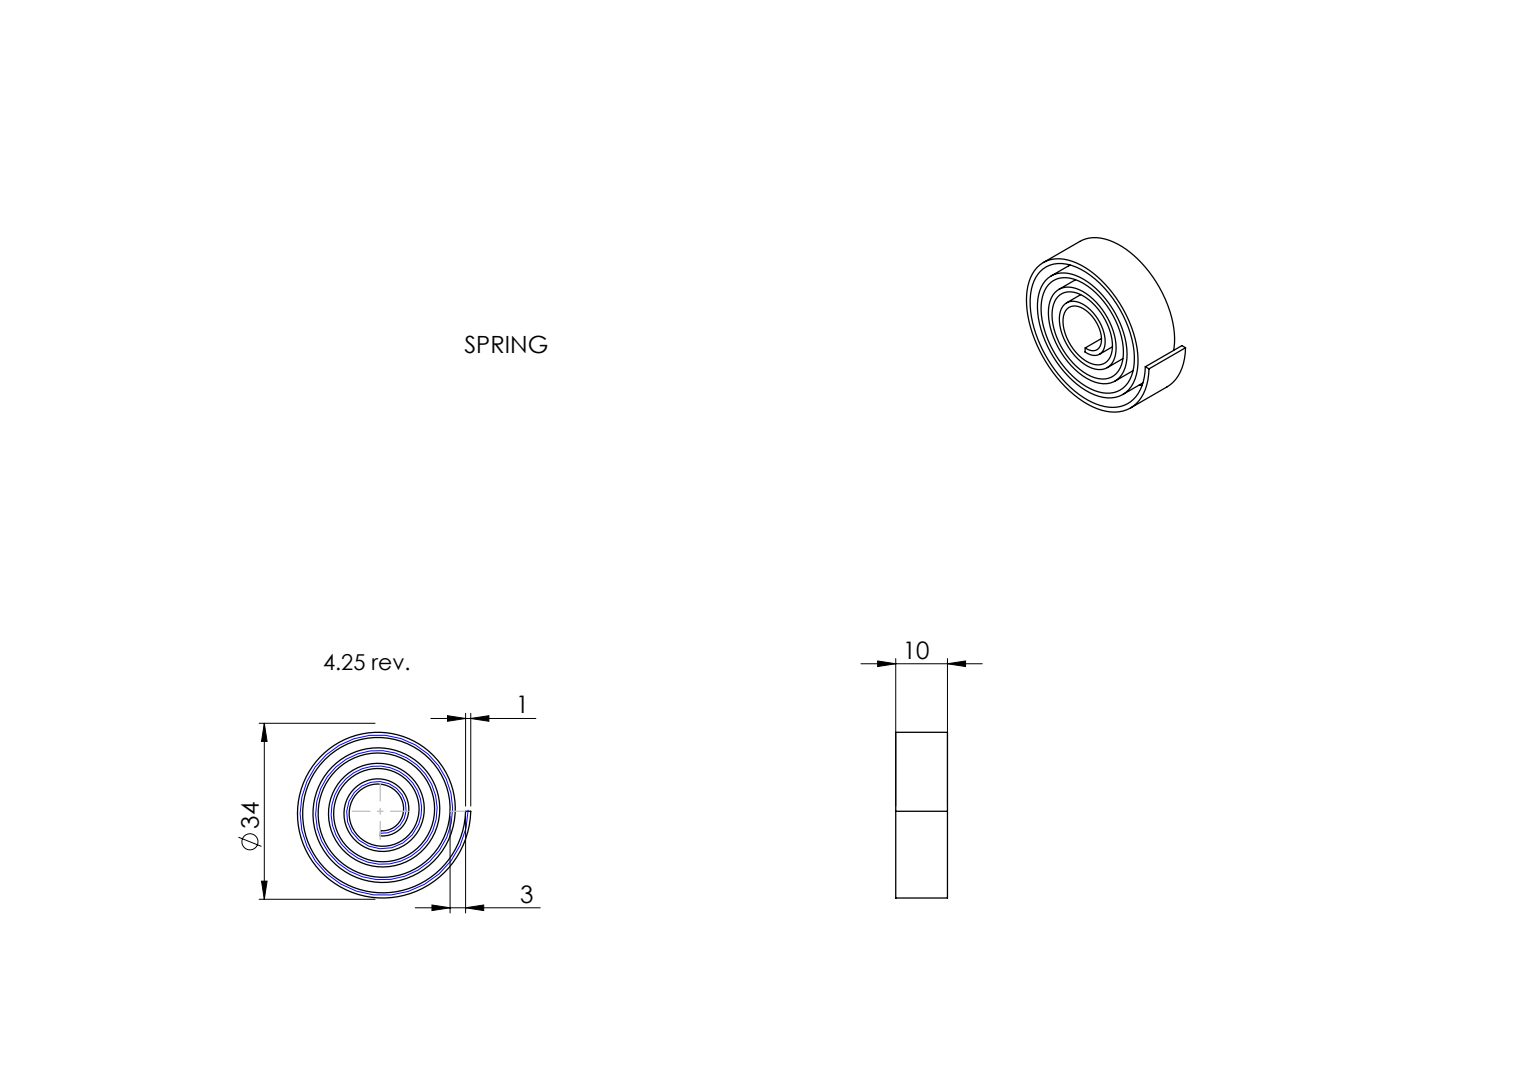
ISO-10303-21;
HEADER;
FILE_DESCRIPTION (('STEP AP214'),
    '1' );
FILE_NAME ('spring.step',
    '2026-10-08T12:30:53',
    ( '' ),
    ( '' ),
    'SwSTEP 2.0',
    'SolidWorks 2026',
    '' );
FILE_SCHEMA (( 'AUTOMOTIVE_DESIGN' ));
ENDSEC;

DATA;
#5=CARTESIAN_POINT ( 'NONE',  ( 13.54728169684850414, 0.8932250400876640128, 10.00000000000000000 ) ) ;
#11=CARTESIAN_POINT ( 'NONE',  ( -13.43906451854578954, -9.301052350413227643, 10.00000000000000000 ) ) ;
#12=CARTESIAN_POINT ( 'NONE',  ( 8.539395351299290837, 0.2748098766782898217, 6.857782953271941950E-17 ) ) ;
#18=PRODUCT ( 'spring', 'spring', '', ( #10456 ) ) ;
#19=EDGE_LOOP ( 'NONE', ( #9760, #9661, #8021, #4048 ) ) ;
#26=CARTESIAN_POINT ( 'NONE',  ( 10.50580257846854337, 1.391709641844861123, 10.00000000000000000 ) ) ;
#31=CARTESIAN_POINT ( 'NONE',  ( 8.800885721068835821, 6.316044917328127895, 3.747395293195558847E-16 ) ) ;
#46=CARTESIAN_POINT ( 'NONE',  ( -11.99326810842395474, 8.590522060507202795, 3.747395293195558847E-16 ) ) ;
#63=CARTESIAN_POINT ( 'NONE',  ( -6.211147023100844322, 2.816369743025010308, 10.00000000000000000 ) ) ;
#73=CARTESIAN_POINT ( 'NONE',  ( 12.88139461472802516, -9.891864711285373701, 10.00000000000000000 ) ) ;
#78=CARTESIAN_POINT ( 'NONE',  ( -3.251399079312189855, 15.05603916236422890, 10.00000000000000000 ) ) ;
#79=CARTESIAN_POINT ( 'NONE',  ( 5.267519402444978738, 2.381954139586884622, 6.857782953271941950E-17 ) ) ;
#88=CARTESIAN_POINT ( 'NONE',  ( -8.694522232909452697, -2.966707450564700643, 10.00000000000000000 ) ) ;
#91=CARTESIAN_POINT ( 'NONE',  ( 9.962304844536467030, 3.945508033568876360, 3.747395293195558847E-16 ) ) ;
#105=CARTESIAN_POINT ( 'NONE',  ( 1.050035089571674352, -12.78847817906846096, 3.747395293195558847E-16 ) ) ;
#109=ORIENTED_EDGE ( 'NONE', *, *, #7807, .F. ) ;
#111=CARTESIAN_POINT ( 'NONE',  ( -10.11701526667144257, 11.92482893257633947, 10.00000000000000000 ) ) ;
#120=CARTESIAN_POINT ( 'NONE',  ( -12.27443204883033623, 3.949650873796764827, 6.857782953271941950E-17 ) ) ;
#127=CARTESIAN_POINT ( 'NONE',  ( -3.043536693350107569, 14.07442491708026111, 10.00000000000000000 ) ) ;
#131=CARTESIAN_POINT ( 'NONE',  ( 10.35108484788239203, -9.702746953904565430, 10.00000000000000000 ) ) ;
#142=CARTESIAN_POINT ( 'NONE',  ( -8.962830026514758686, 0.7152994853347287574, 10.00000000000000000 ) ) ;
#146=CARTESIAN_POINT ( 'NONE',  ( -0.1586286459269546645, 8.284426055182338544, 3.747395293195558847E-16 ) ) ;
#147=CARTESIAN_POINT ( 'NONE',  ( -14.12277927129995803, -8.146689865454474599, 6.857782953271941950E-17 ) ) ;
#160=CARTESIAN_POINT ( 'NONE',  ( 4.123629756449401107, -15.38522696314584515, 3.747395293195558847E-16 ) ) ;
#161=B_SPLINE_CURVE_WITH_KNOTS ( 'NONE', 3,
 ( #5386, #11258, #9477, #10271, #12042, #10215, #12099, #7452, #5566, #5686, #3851, #160, #7515, #4646, #6654, #11313, #9416, #9236, #7383, #10392, #2746, #1763, #2872, #3726, #5623, #6594, #5504, #8321, #3906, #856, #2009, #46, #11199, #4589, #1040, #5753, #1094, #913, #4825, #7630, #10329, #8563, #2815, #11374, #6539, #2994, #9353, #6716, #3663, #11126, #7571, #6477, #4770, #1830, #9296, #3796, #1889, #970, #8381, #4710, #8449, #1947, #8509, #2933, #105, #5808, #11490, #10452, #2070, #5004, #9535, #1151, #7935, #4206, #2189, #4887, #8625, #2303, #3969, #3113, #8687, #225, #10574, #5125, #8800, #6946, #5984, #7698, #11433, #6039, #1391, #1325, #4087, #10690, #4024, #9597, #3053, #3228, #6772, #10509, #9711, #1215, #9768, #2124, #5062, #8863, #11664, #408, #7880, #5865, #4951, #3282, #6828, #5928, #468, #286, #7753, #9657, #1271, #4153, #8742, #2249, #11611, #345, #7815, #11553, #3175, #6894, #10638, #8975, #3350, #11847, #7002, #11906, #8058, #9153, #10749, #585, #7066, #6106, #3533, #7247, #11790, #770, #2367, #4324, #10820, #9840, #11001, #2551, #1450, #528, #2615, #7987, #11723, #8178, #11967, #4444, #2429, #3420, #4261, #4507, #5185, #6350, #5309, #7127, #8920, #10933, #10073, #1692, #6167, #5425, #8243, #4388, #10877, #9895, #7186, #1508, #5243, #2488, #6225, #9952, #1569, #9100, #9042, #6290, #655, #8121, #3476, #10010, #1636, #5374, #710, #8306, #12028, #6526, #1933, #2735, #5669, #3652, #6463, #3595, #7435, #11056, #2671, #7560, #3838, #4633 ),
 .UNSPECIFIED., .F., .F.,
 ( 4, 2, 2, 2, 2, 2, 2, 2, 2, 2, 2, 2, 2, 2, 2, 2, 2, 2, 2, 2, 2, 2, 2, 2, 2, 2, 2, 2, 2, 2, 2, 2, 2, 2, 2, 2, 2, 2, 2, 2, 2, 2, 2, 2, 2, 2, 2, 2, 2, 2, 2, 2, 2, 2, 2, 2, 2, 2, 2, 2, 2, 2, 2, 2, 2, 2, 2, 2, 2, 2, 2, 2, 2, 2, 2, 2, 2, 2, 2, 2, 2, 2, 2, 2, 2, 2, 2, 2, 2, 2, 2, 2, 2, 2, 2, 2, 2, 2, 2, 2, 2, 2, 2, 4 ),
 ( 0.000000000000000000, 0.007812500000000000000, 0.01562500000000000000, 0.02343750000000000000, 0.03125000000000000000, 0.03906250000000000000, 0.04687500000000000000, 0.05468750000000000000, 0.06250000000000000000, 0.07031250000000000000, 0.07812500000000000000, 0.08593750000000000000, 0.09375000000000000000, 0.1015624999999999861, 0.1093750000000000000, 0.1171875000000000000, 0.1250000000000000000, 0.1328125000000000000, 0.1406250000000000000, 0.1484375000000000000, 0.1562500000000000000, 0.1640624999999999722, 0.1718750000000000000, 0.1796875000000000000, 0.1875000000000000000, 0.1953125000000000000, 0.2031249999999999722, 0.2109375000000000000, 0.2187500000000000000, 0.2265625000000000000, 0.2343750000000000000, 0.2421875000000000000, 0.2500000000000000000, 0.2578125000000000000, 0.2656250000000000000, 0.2734375000000000000, 0.2812500000000000000, 0.2890625000000000000, 0.2968750000000000000, 0.3046875000000000000, 0.3125000000000000000, 0.3203125000000000000, 0.3281249999999999445, 0.3359375000000000000, 0.3437500000000000000, 0.3515625000000000000, 0.3593750000000000000, 0.3671874999999999445, 0.3750000000000000000, 0.3828125000000000000, 0.3906250000000000000, 0.3984375000000000000, 0.4062499999999999445, 0.4140625000000000000, 0.4218750000000000000, 0.4296875000000000000, 0.4375000000000000000, 0.4453125000000000000, 0.4531250000000000000, 0.4609375000000000000, 0.4687500000000000000, 0.4765625000000000000, 0.4843750000000000000, 0.4921875000000000000, 0.5000000000000000000, 0.5078125000000000000, 0.5156250000000000000, 0.5234375000000000000, 0.5312500000000000000, 0.5390625000000000000, 0.5468750000000000000, 0.5546875000000000000, 0.5625000000000000000, 0.5703125000000000000, 0.5781250000000000000, 0.5859375000000000000, 0.5937500000000000000, 0.6015625000000000000, 0.6093750000000000000, 0.6171874999999998890, 0.6250000000000000000, 0.6328125000000000000, 0.6406250000000000000, 0.6484375000000000000, 0.6562499999999998890, 0.6640625000000000000, 0.6718750000000000000, 0.6796875000000000000, 0.6875000000000000000, 0.6953124999999998890, 0.7031250000000000000, 0.7109375000000000000, 0.7187500000000000000, 0.7265625000000000000, 0.7343749999999998890, 0.7421875000000000000, 0.7500000000000000000, 0.7656250000000000000, 0.7812500000000000000, 0.7968750000000000000, 0.8124999999999998890, 0.8281250000000000000, 0.8437500000000000000, 0.8499999999999999778 ),
 .UNSPECIFIED. ) ;
#167=CARTESIAN_POINT ( 'NONE',  ( -12.80690425020244128, 9.177692349400032867, 10.00000000000000000 ) ) ;
#177=CARTESIAN_POINT ( 'NONE',  ( -10.84705874452746066, 6.751620637727320684, 6.857782953271941950E-17 ) ) ;
#185=CARTESIAN_POINT ( 'NONE',  ( -15.00596061316374197, -1.728743269517114767, 10.00000000000000000 ) ) ;
#191=CARTESIAN_POINT ( 'NONE',  ( 14.53830338343600559, -0.2437330612273629071, 10.00000000000000000 ) ) ;
#202=CARTESIAN_POINT ( 'NONE',  ( 2.581500635392915299, -6.456130005640037695, 10.00000000000000000 ) ) ;
#206=CARTESIAN_POINT ( 'NONE',  ( 7.605204090344414247, 4.385345779697003010, 10.00000000000000000 ) ) ;
#208=CARTESIAN_POINT ( 'NONE',  ( -12.06849956494802889, -5.462025159506374017, 6.857782953271941950E-17 ) ) ;
#213=EDGE_CURVE ( 'NONE', #1474, #6584, #2468, .T. ) ;
#225=CARTESIAN_POINT ( 'NONE',  ( -10.51222845931327576, 5.388985543800765221, 3.747395293195558847E-16 ) ) ;
#233=CARTESIAN_POINT ( 'NONE',  ( 4.382127860174852785, -16.35473703246191235, 10.00000000000000000 ) ) ;
#244=CARTESIAN_POINT ( 'NONE',  ( 5.334478431285537781, 14.15651896542076749, 6.857782953271941950E-17 ) ) ;
#252=CARTESIAN_POINT ( 'NONE',  ( -4.793139000956300855, -14.90149022103883247, 10.00000000000000000 ) ) ;
#259=CARTESIAN_POINT ( 'NONE',  ( 7.737545192982512532, 9.111483571581279861, 10.00000000000000000 ) ) ;
#262=CARTESIAN_POINT ( 'NONE',  ( -6.423942855642367000, 13.01866063961475461, 3.747395293195558847E-16 ) ) ;
#270=CARTESIAN_POINT ( 'NONE',  ( 1.482756436301465808, -6.713508106970953015, 10.00000000000000000 ) ) ;
#272=CARTESIAN_POINT ( 'NONE',  ( 11.51680056346192593, -0.3781118375584788249, 10.00000000000000000 ) ) ;
#273=CARTESIAN_POINT ( 'NONE',  ( 1.748316258820581170, 15.14524454193558611, 6.857782953271941950E-17 ) ) ;
#281=CARTESIAN_POINT ( 'NONE',  ( 3.017784444055084503, -16.62017357425735753, 6.857782953271941950E-17 ) ) ;
#286=CARTESIAN_POINT ( 'NONE',  ( 0.6578947103914138950, -9.792230064638470566, 3.747395293195558847E-16 ) ) ;
#293=CARTESIAN_POINT ( 'NONE',  ( -15.56595607421884075, -4.438723023272252988, 10.00000000000000000 ) ) ;
#305=CARTESIAN_POINT ( 'NONE',  ( -3.251399079312188078, 15.05603916236422180, 6.857782953271941950E-17 ) ) ;
#312=CARTESIAN_POINT ( 'NONE',  ( 4.071483724746832067, 10.33449570568845211, 10.00000000000000000 ) ) ;
#314=( NAMED_UNIT ( * ) PLANE_ANGLE_UNIT ( ) SI_UNIT ( $, .RADIAN. ) );
#317=CARTESIAN_POINT ( 'NONE',  ( 12.58137556868281237, 7.823023050435613968, 10.00000000000000000 ) ) ;
#329=CARTESIAN_POINT ( 'NONE',  ( -0.7379871813790722657, -6.677365878963855472, 10.00000000000000000 ) ) ;
#333=CARTESIAN_POINT ( 'NONE',  ( -8.201440678128605555, 5.289679325232168772, 10.00000000000000000 ) ) ;
#334=CARTESIAN_POINT ( 'NONE',  ( -15.59049818040117152, 3.373450308083002724, 6.857782953271941950E-17 ) ) ;
#342=CARTESIAN_POINT ( 'NONE',  ( 7.795318149608632119, -14.02504990430958998, 10.00000000000000000 ) ) ;
#345=CARTESIAN_POINT ( 'NONE',  ( -7.402161455537873636, -5.702533393948970186, 3.747395293195558847E-16 ) ) ;
#349=CARTESIAN_POINT ( 'NONE',  ( 17.46093749967478814, -1.431715403549062904, 10.00000000000000000 ) ) ;
#352=VECTOR ( 'NONE', #8492, 1000.000000000000000 ) ;
#359=CARTESIAN_POINT ( 'NONE',  ( -2.240087900411201982, -13.53314956822677928, 6.857782953271941950E-17 ) ) ;
#369=CARTESIAN_POINT ( 'NONE',  ( -4.046710180314750716, 10.72208681399755648, 10.00000000000000000 ) ) ;
#377=CARTESIAN_POINT ( 'NONE',  ( 2.259453438922059298, -13.68937604509904737, 10.00000000000000000 ) ) ;
#379=CARTESIAN_POINT ( 'NONE',  ( -11.21689850597007343, 9.520844388990626683, 3.747395293195558847E-16 ) ) ;
#391=CARTESIAN_POINT ( 'NONE',  ( -6.589974825828277538, 7.038139701356666222, 10.00000000000000000 ) ) ;
#393=CARTESIAN_POINT ( 'NONE',  ( -12.72059027619867244, -3.407653011835690471, 6.857782953271941950E-17 ) ) ;
#408=CARTESIAN_POINT ( 'NONE',  ( 8.913847851857145344, -5.129921849437907078, 3.747395293195558847E-16 ) ) ;
#413=CARTESIAN_POINT ( 'NONE',  ( -8.799721882313775723, 9.100398320382247164, 10.00000000000000000 ) ) ;
#424=CARTESIAN_POINT ( 'NONE',  ( -9.352287007201468327, 3.176141031410556703, 6.857782953271941950E-17 ) ) ;
#430=CARTESIAN_POINT ( 'NONE',  ( -8.984113827416489784, -1.502549133976348816, 10.00000000000000000 ) ) ;
#439=CARTESIAN_POINT ( 'NONE',  ( 3.343943643650761022, -10.41127694127790271, 10.00000000000000000 ) ) ;
#454=CARTESIAN_POINT ( 'NONE',  ( 5.893263639827395650, 6.717612500730409941, 10.00000000000000000 ) ) ;
#456=CARTESIAN_POINT ( 'NONE',  ( 5.343773788080180331, 10.82393792025543711, 6.857782953271941950E-17 ) ) ;
#468=CARTESIAN_POINT ( 'NONE',  ( 2.257301671556970479, -9.631158585656898197, 3.747395293195558847E-16 ) ) ;
#473=CARTESIAN_POINT ( 'NONE',  ( 14.27634331491212549, 3.322769473269123974, 10.00000000000000000 ) ) ;
#485=CARTESIAN_POINT ( 'NONE',  ( -8.201440678127905670, 5.289679325232165219, 6.857782953271941950E-17 ) ) ;
#491=CARTESIAN_POINT ( 'NONE',  ( -10.00031051369627200, 6.213292778947749007, 10.00000000000000000 ) ) ;
#498=CARTESIAN_POINT ( 'NONE',  ( -4.368568794346924022, -9.638580752213403713, 10.00000000000000000 ) ) ;
#500=CARTESIAN_POINT ( 'NONE',  ( -11.74902089294173457, -3.156991809147609906, 3.747395293195558847E-16 ) ) ;
#513=CARTESIAN_POINT ( 'NONE',  ( 2.919619825260427071, -7.400844473264730716, 10.00000000000000000 ) ) ;
#514=CARTESIAN_POINT ( 'NONE',  ( -3.909826107002860596, 8.641065831729461522, 6.857782953271941950E-17 ) ) ;
#522=CARTESIAN_POINT ( 'NONE',  ( -15.00596061316374197, -1.728743269517114767, 10.00000000000000000 ) ) ;
#528=CARTESIAN_POINT ( 'NONE',  ( 7.195390336726608105, 2.736402267197653337, 3.747395293195558847E-16 ) ) ;
#533=CARTESIAN_POINT ( 'NONE',  ( -11.61414229320030778, -6.453515506896109422, 10.00000000000000000 ) ) ;
#543=CARTESIAN_POINT ( 'NONE',  ( -3.909826107002860596, 8.641065831729461522, 6.857782953271941950E-17 ) ) ;
#550=CARTESIAN_POINT ( 'NONE',  ( 8.800885721068839374, 6.316044917328129671, 10.00000000000000000 ) ) ;
#558=CARTESIAN_POINT ( 'NONE',  ( 0.7062845326068618590, -10.79445016380499212, 10.00000000000000000 ) ) ;
#560=CARTESIAN_POINT ( 'NONE',  ( 7.972781652389871354, 11.51689705412852405, 3.747395293195558847E-16 ) ) ;
#575=CARTESIAN_POINT ( 'NONE',  ( 2.798030692818294085, 8.692477993603722197, 6.857782953271941950E-17 ) ) ;
#582=CARTESIAN_POINT ( 'NONE',  ( -14.24631147015002242, -5.364320868108786833, 10.00000000000000000 ) ) ;
#585=CARTESIAN_POINT ( 'NONE',  ( -4.158289900079266133, 7.437556212723415605, 3.747395293195558847E-16 ) ) ;
#595=CARTESIAN_POINT ( 'NONE',  ( -5.414455899168761022, -12.47541146649038879, 10.00000000000000000 ) ) ;
#608=CARTESIAN_POINT ( 'NONE',  ( -7.708066421255707290, 5.920849505456867945, 6.857782953271941950E-17 ) ) ;
#617=CARTESIAN_POINT ( 'NONE',  ( 5.657123057053187409, 5.504982807385219168, 10.00000000000000000 ) ) ;
#625=CARTESIAN_POINT ( 'NONE',  ( 7.252227276002106038, 5.017415995114419047, 10.00000000000000000 ) ) ;
#628=CARTESIAN_POINT ( 'NONE',  ( -1.035167565893234443, -12.71157708251009133, 3.747395293195558847E-16 ) ) ;
#640=CARTESIAN_POINT ( 'NONE',  ( 1.661435237661583297, -7.700870200009183542, 10.00000000000000000 ) ) ;
#641=CARTESIAN_POINT ( 'NONE',  ( -4.625218816436122538, 8.325684435358754243, 6.857782953271941950E-17 ) ) ;
#650=CARTESIAN_POINT ( 'NONE',  ( -2.069312577552833154, -12.54440658741724235, 10.00000000000000000 ) ) ;
#654=CARTESIAN_POINT ( 'NONE',  ( 0.03696586647634111239, -4.250492970015663730, 10.00000000000000000 ) ) ;
#655=CARTESIAN_POINT ( 'NONE',  ( -4.158472309566738190, 3.840014155104740201, 3.747395293195558847E-16 ) ) ;
#663=CARTESIAN_POINT ( 'NONE',  ( -1.784247137544766604, 5.123456263349899231, 10.00000000000000000 ) ) ;
#671=CARTESIAN_POINT ( 'NONE',  ( 10.96671743108978525, -3.132869264233209439, 6.857782953271941950E-17 ) ) ;
#677=CARTESIAN_POINT ( 'NONE',  ( 7.536008357046525497, 0.2705779428718255719, 10.00000000000000000 ) ) ;
#685=CARTESIAN_POINT ( 'NONE',  ( -0.2556890074706391625, -7.756263830888999067, 10.00000000000000000 ) ) ;
#692=CARTESIAN_POINT ( 'NONE',  ( 6.411932913580776550, 4.469049885107575726, 3.747395293195558847E-16 ) ) ;
#698=CARTESIAN_POINT ( 'NONE',  ( -6.211147023100844322, 2.816369743025010308, 10.00000000000000000 ) ) ;
#699=CARTESIAN_POINT ( 'NONE',  ( -8.665663522307772482, -5.581295667939712324, 6.857782953271941950E-17 ) ) ;
#706=CARTESIAN_POINT ( 'NONE',  ( -5.318373871714366707, 13.46535835423756566, 10.00000000000000000 ) ) ;
#710=CARTESIAN_POINT ( 'NONE',  ( -0.4771094043438768861, 5.286185534804329400, 3.747395293195558847E-16 ) ) ;
#724=CARTESIAN_POINT ( 'NONE',  ( 7.763517025772753044, -3.069710483245351451, 6.857782953271941950E-17 ) ) ;
#731=CARTESIAN_POINT ( 'NONE',  ( 6.723006375386864519, 3.907299473125435796, 10.00000000000000000 ) ) ;
#739=CARTESIAN_POINT ( 'NONE',  ( 17.46093749967478104, -1.431715403549062460, 6.857782953271941950E-17 ) ) ;
#746=ADVANCED_FACE ( 'NONE', ( #3811 ), #3925, .T. ) ;
#749=CARTESIAN_POINT ( 'NONE',  ( 0.8073695008816142993, 5.181225205791315958, 3.747395293195558847E-16 ) ) ;
#750=AXIS2_PLACEMENT_3D ( 'NONE', #910, #10269, #9233 ) ;
#756=CARTESIAN_POINT ( 'NONE',  ( 2.529667540517110513, -4.392173529266737653, 10.00000000000000000 ) ) ;
#757=CARTESIAN_POINT ( 'NONE',  ( 4.138106518798946531, 8.052838533163340529, 6.857782953271941950E-17 ) ) ;
#763=CARTESIAN_POINT ( 'NONE',  ( -8.499083411061075566, 11.86528080735166490, 10.00000000000000000 ) ) ;
#770=CARTESIAN_POINT ( 'NONE',  ( 1.831757423467612389, 7.960349185506225389, 3.747395293195558847E-16 ) ) ;
#794=CARTESIAN_POINT ( 'NONE',  ( 7.195390336726611658, 2.736402267197346028, 10.00000000000000000 ) ) ;
#803=CARTESIAN_POINT ( 'NONE',  ( 3.017784444055084503, -16.62017357425735753, 6.857782953271941950E-17 ) ) ;
#809=ORIENTED_EDGE ( 'NONE', *, *, #6284, .T. ) ;
#813=CARTESIAN_POINT ( 'NONE',  ( 7.527773320476327079, 0.8933511214758176333, 3.747395293195558847E-16 ) ) ;
#822=CARTESIAN_POINT ( 'NONE',  ( 2.529667540516381319, -4.392173529266732324, 6.857782953271941950E-17 ) ) ;
#832=CARTESIAN_POINT ( 'NONE',  ( -10.00031051369627200, 6.213292778947749007, 10.00000000000000000 ) ) ;
#838=CARTESIAN_POINT ( 'NONE',  ( -3.937910939466568117, -8.732312745279397603, 3.747395293195558847E-16 ) ) ;
#852=UNCERTAINTY_MEASURE_WITH_UNIT (LENGTH_MEASURE( 1.000000000000000082E-05 ), #3873, 'distance_accuracy_value', 'NONE');
#856=CARTESIAN_POINT ( 'NONE',  ( -13.83044629298881034, 5.462350471645222250, 3.747395293195558847E-16 ) ) ;
#857=CARTESIAN_POINT ( 'NONE',  ( 8.393308867179008814, -1.106660293010312213, 6.857782953271941950E-17 ) ) ;
#865=CARTESIAN_POINT ( 'NONE',  ( -3.432991321284830200, 4.402131891631372973, 10.00000000000000000 ) ) ;
#872=CARTESIAN_POINT ( 'NONE',  ( -5.542557460684662374, -4.854674288180239827, 10.00000000000000000 ) ) ;
#880=CARTESIAN_POINT ( 'NONE',  ( -0.7379871813790714885, -6.677365878963852808, 3.747395293195558847E-16 ) ) ;
#885=CARTESIAN_POINT ( 'NONE',  ( 4.382127860174852785, -16.35473703246191235, 10.00000000000000000 ) ) ;
#886=CARTESIAN_POINT ( 'NONE',  ( 0.3111040546027372677, -4.780743156735971944, 6.857782953271941950E-17 ) ) ;
#892=CARTESIAN_POINT ( 'NONE',  ( 4.071483724746832067, 10.33449570568845211, 10.00000000000000000 ) ) ;
#897=CARTESIAN_POINT ( 'NONE',  ( 10.00611923916670953, -2.842981073525689517, 3.747395293195558847E-16 ) ) ;
#910=CARTESIAN_POINT ( 'NONE',  ( 17.49999999999999645, 0.000000000000000000, 6.857782953271941950E-17 ) ) ;
#913=CARTESIAN_POINT ( 'NONE',  ( -3.043536693350106681, 14.07442491708025756, 3.747395293195558847E-16 ) ) ;
#914=CARTESIAN_POINT ( 'NONE',  ( -6.191802569540376666, -3.848120238389427072, 6.857782953271941950E-17 ) ) ;
#926=CARTESIAN_POINT ( 'NONE',  ( -4.263796145714478847, -6.152586724582791433, 10.00000000000000000 ) ) ;
#936=CARTESIAN_POINT ( 'NONE',  ( -4.158472309566738190, 3.840014155104740201, 3.747395293195558847E-16 ) ) ;
#942=CARTESIAN_POINT ( 'NONE',  ( 17.24531215409499296, -2.853661713830125013, 10.00000000000000000 ) ) ;
#943=CARTESIAN_POINT ( 'NONE',  ( 5.893263639826756162, 6.717612500731040548, 6.857782953271941950E-17 ) ) ;
#951=CARTESIAN_POINT ( 'NONE',  ( 10.39479819782869896, 2.258419626871297492, 10.00000000000000000 ) ) ;
#955=CARTESIAN_POINT ( 'NONE',  ( 1.454091968623351327, 11.13059540125182423, 3.747395293195558847E-16 ) ) ;
#970=CARTESIAN_POINT ( 'NONE',  ( 10.36190401370965475, -8.216093097539266310, 3.747395293195558847E-16 ) ) ;
#971=CARTESIAN_POINT ( 'NONE',  ( 1.022653496104248605, 6.171874473422422902, 6.857782953271941950E-17 ) ) ;
#989=CARTESIAN_POINT ( 'NONE',  ( 17.24531215409252383, -2.853661713830123237, 6.857782953271941950E-17 ) ) ;
#990=CARTESIAN_POINT ( 'NONE',  ( 0.0002901587068754535662, -4.749354241797641762, 5.000000000000000000 ) ) ;
#999=CARTESIAN_POINT ( 'NONE',  ( 4.163410377374356486, -12.26152398776834396, 10.00000000000000000 ) ) ;
#1008=CARTESIAN_POINT ( 'NONE',  ( -6.864300873105356082, 13.92024697337932082, 10.00000000000000000 ) ) ;
#1009=CARTESIAN_POINT ( 'NONE',  ( -6.211147023100837217, 2.816369743025007644, 6.857782953271941950E-17 ) ) ;
#1021=CARTESIAN_POINT ( 'NONE',  ( -10.51222845931418703, 5.388985543801221745, 10.00000000000000000 ) ) ;
#1024=CARTESIAN_POINT ( 'NONE',  ( -6.925491926711623059, 5.292860106065907289, 3.747395293195558847E-16 ) ) ;
#1040=CARTESIAN_POINT ( 'NONE',  ( -8.499083411061073789, 11.86528080735276269, 3.747395293195558847E-16 ) ) ;
#1045=CARTESIAN_POINT ( 'NONE',  ( -1.103316172498668202, -16.73802372459124754, 10.00000000000000000 ) ) ;
#1053=CARTESIAN_POINT ( 'NONE',  ( 4.479449988082533807, -13.21383449271837840, 6.857782953271941950E-17 ) ) ;
#1062=CARTESIAN_POINT ( 'NONE',  ( -6.423942855642368777, 13.01866063961585951, 10.00000000000000000 ) ) ;
#1069=CARTESIAN_POINT ( 'NONE',  ( -4.384918567263696332, -12.91535881965571342, 10.00000000000000000 ) ) ;
#1077=CARTESIAN_POINT ( 'NONE',  ( 10.41236255589547177, -1.188820951657899361, 10.00000000000000000 ) ) ;
#1079=CARTESIAN_POINT ( 'NONE',  ( -8.409270314015810044, 2.833341551407462244, 3.747395293195558847E-16 ) ) ;
#1080=CARTESIAN_POINT ( 'NONE',  ( -14.19814495527598730, 7.008511237308412412, 6.857782953271941950E-17 ) ) ;
#1094=CARTESIAN_POINT ( 'NONE',  ( -5.318373871714365819, 13.46535835423756389, 3.747395293195558847E-16 ) ) ;
#1107=CARTESIAN_POINT ( 'NONE',  ( -9.546882484473291797, 8.373557015400844961, 6.857782953271941950E-17 ) ) ;
#1114=CARTESIAN_POINT ( 'NONE',  ( 11.62709622633371076, -6.461356448465072511, 10.00000000000000000 ) ) ;
#1121=CARTESIAN_POINT ( 'NONE',  ( -6.266017822847497420, 10.86399168115691438, 10.00000000000000000 ) ) ;
#1123=CARTESIAN_POINT ( 'NONE',  ( -14.24631147015001886, -5.364320868109360596, 3.747395293195558847E-16 ) ) ;
#1133=CARTESIAN_POINT ( 'NONE',  ( 7.402789038520873000, -0.9464297003978345835, 10.00000000000000000 ) ) ;
#1135=CARTESIAN_POINT ( 'NONE',  ( -9.977213461302319786, -1.645879626164742593, 10.00000000000000000 ) ) ;
#1137=CARTESIAN_POINT ( 'NONE',  ( -4.384918567263694555, -12.91535881965570631, 6.857782953271941950E-17 ) ) ;
#1151=CARTESIAN_POINT ( 'NONE',  ( -9.045553118584754415, -8.482981269326389295, 3.747395293195558847E-16 ) ) ;
#1156=CARTESIAN_POINT ( 'NONE',  ( -14.19814495527487352, 7.008511237308415964, 10.00000000000000000 ) ) ;
#1165=CARTESIAN_POINT ( 'NONE',  ( 2.259453438922057522, -13.68937604509904027, 6.857782953271941950E-17 ) ) ;
#1173=CARTESIAN_POINT ( 'NONE',  ( 13.24268851590354146, -2.403973981685017414, 10.00000000000000000 ) ) ;
#1178=CARTESIAN_POINT ( 'NONE',  ( 9.056240860197965148, 7.682302481599247557, 10.00000000000000000 ) ) ;
#1181=CARTESIAN_POINT ( 'NONE',  ( 6.600721363681633314, -14.58171973507987396, 3.747395293195558847E-16 ) ) ;
#1191=CARTESIAN_POINT ( 'NONE',  ( -4.428608208598376450, -4.627450663479480752, 10.00000000000000000 ) ) ;
#1197=CARTESIAN_POINT ( 'NONE',  ( 8.235329212248927888, -1.783486464602662691, 10.00000000000000000 ) ) ;
#1198=CARTESIAN_POINT ( 'NONE',  ( -5.683926142426733108, 14.39978054689283660, 6.857782953271941950E-17 ) ) ;
#1215=CARTESIAN_POINT ( 'NONE',  ( 10.39479819782869541, 2.258419626871296604, 3.747395293195558847E-16 ) ) ;
#1221=CARTESIAN_POINT ( 'NONE',  ( -15.85416723795449556, 2.087521067385502693, 10.00000000000000000 ) ) ;
#1231=CARTESIAN_POINT ( 'NONE',  ( 10.35108484788238670, -9.702746953904560101, 6.857782953271941950E-17 ) ) ;
#1240=CARTESIAN_POINT ( 'NONE',  ( 10.50580257846854337, 1.391709641844861123, 10.00000000000000000 ) ) ;
#1244=( NAMED_UNIT ( * ) SI_UNIT ( $, .STERADIAN. ) SOLID_ANGLE_UNIT ( ) );
#1249=CARTESIAN_POINT ( 'NONE',  ( 13.14573027368779456, 6.745762002080610387, 10.00000000000000000 ) ) ;
#1252=CARTESIAN_POINT ( 'NONE',  ( 2.839002905303027013, -15.63284973865750693, 3.747395293195558847E-16 ) ) ;
#1259=CARTESIAN_POINT ( 'NONE',  ( 7.195390336726611658, 2.736402267197346028, 10.00000000000000000 ) ) ;
#1261=CARTESIAN_POINT ( 'NONE',  ( -9.650762677556034674, -3.270672451565360461, 10.00000000000000000 ) ) ;
#1262=CARTESIAN_POINT ( 'NONE',  ( 7.619603487155711008, -11.82824555707797387, 6.857782953271941950E-17 ) ) ;
#1271=CARTESIAN_POINT ( 'NONE',  ( -2.487495860704069361, -9.331140650584718088, 3.747395293195558847E-16 ) ) ;
#1279=CARTESIAN_POINT ( 'NONE',  ( -14.76245309360257174, 5.834016798581408203, 10.00000000000000000 ) ) ;
#1288=CARTESIAN_POINT ( 'NONE',  ( -12.80690425020131684, 9.177692349400029315, 6.857782953271941950E-17 ) ) ;
#1295=CARTESIAN_POINT ( 'NONE',  ( 0.6578947103914143391, -9.792230064638474119, 10.00000000000000000 ) ) ;
#1300=CARTESIAN_POINT ( 'NONE',  ( 14.22875512193219372, -2.589574901423981501, 10.00000000000000000 ) ) ;
#1312=CARTESIAN_POINT ( 'NONE',  ( -9.352287007200070335, 3.176141031410558924, 10.00000000000000000 ) ) ;
#1313=CARTESIAN_POINT ( 'NONE',  ( -8.739072045530900112, -14.04184524613900820, 6.857782953271941950E-17 ) ) ;
#1325=CARTESIAN_POINT ( 'NONE',  ( 1.454091968623351327, 11.13059540125182423, 3.747395293195558847E-16 ) ) ;
#1331=CARTESIAN_POINT ( 'NONE',  ( -12.98359546555290045, 0.8565524458112724338, 10.00000000000000000 ) ) ;
#1344=CARTESIAN_POINT ( 'NONE',  ( -1.916691774771271284, -10.52688368019216014, 6.857782953271941950E-17 ) ) ;
#1351=CARTESIAN_POINT ( 'NONE',  ( -7.812220363924760491, -5.053636123081433951, 10.00000000000000000 ) ) ;
#1355=SURFACE_SIDE_STYLE ('',( #9737 ) ) ;
#1359=CARTESIAN_POINT ( 'NONE',  ( 7.334967666341840165, -8.371827447635059372, 10.00000000000000000 ) ) ;
#1361=CARTESIAN_POINT ( 'NONE',  ( 11.04976219204102783, -11.79656285006036676, 3.747395293195558847E-16 ) ) ;
#1375=CARTESIAN_POINT ( 'NONE',  ( 2.084091085258986897, 8.931495281877387171, 10.00000000000000000 ) ) ;
#1376=CARTESIAN_POINT ( 'NONE',  ( 2.469054641153893837, -10.61194774715159284, 6.857782953271941950E-17 ) ) ;
#1391=CARTESIAN_POINT ( 'NONE',  ( -0.3758430365714711674, 11.29677535215814110, 3.747395293195558847E-16 ) ) ;
#1398=CARTESIAN_POINT ( 'NONE',  ( 11.20109743375192224, 9.815261043520028039, 10.00000000000000000 ) ) ;
#1408=CARTESIAN_POINT ( 'NONE',  ( 7.605204090343169909, 4.385345779697310320, 6.857782953271941950E-17 ) ) ;
#1415=CARTESIAN_POINT ( 'NONE',  ( -11.32214898804313208, 3.633524203737720448, 10.00000000000000000 ) ) ;
#1422=CARTESIAN_POINT ( 'NONE',  ( 4.764169229607557732, 7.652272242165495619, 10.00000000000000000 ) ) ;
#1424=CARTESIAN_POINT ( 'NONE',  ( 5.172292865810426576, -11.91455349003027564, 3.747395293195558847E-16 ) ) ;
#1438=CARTESIAN_POINT ( 'NONE',  ( 5.508953106497951779, 1.454581011951755043, 10.00000000000000000 ) ) ;
#1439=CARTESIAN_POINT ( 'NONE',  ( 7.334967666341834835, -8.371827447635054043, 6.857782953271941950E-17 ) ) ;
#1446=CARTESIAN_POINT ( 'NONE',  ( -1.872083171988683015, 14.23747171912756393, 10.00000000000000000 ) ) ;
#1450=CARTESIAN_POINT ( 'NONE',  ( 6.723006375386860967, 3.907299473125124489, 3.747395293195558847E-16 ) ) ;
#1456=CARTESIAN_POINT ( 'NONE',  ( -12.72059027619867955, -3.407653011836159873, 10.00000000000000000 ) ) ;
#1467=CARTESIAN_POINT ( 'NONE',  ( -8.209791827104812256, -6.297951179201748850, 6.857782953271941950E-17 ) ) ;
#1473=CARTESIAN_POINT ( 'NONE',  ( -3.141381368647836236, 10.98006565327106543, 10.00000000000000000 ) ) ;
#1474=VERTEX_POINT ( 'NONE', #5660 ) ;
#1481=CARTESIAN_POINT ( 'NONE',  ( 6.242895496889244278, -5.302832405932367266, 10.00000000000000000 ) ) ;
#1483=CARTESIAN_POINT ( 'NONE',  ( 13.29800827116429573, 3.099979537169514909, 3.747395293195558847E-16 ) ) ;
#1497=CARTESIAN_POINT ( 'NONE',  ( -9.977213461302312680, -1.645879626164740817, 6.857782953271941950E-17 ) ) ;
#1498=CARTESIAN_POINT ( 'NONE',  ( 17.49999999999999645, 0.000000000000000000, 6.857782953271941950E-17 ) ) ;
#1503=CARTESIAN_POINT ( 'NONE',  ( 1.050035089571674352, -12.78847817906846451, 10.00000000000000000 ) ) ;
#1507=B_SPLINE_CURVE_WITH_KNOTS ( 'NONE', 3,
 ( #9651, #11485, #8796, #2183, #3107, #6769, #6824, #10566, #3170, #342, #6942, #10633, #9834, #11660, #3277, #4881, #8916, #1632, #5421, #4503, #6283, #3590, #8116, #582, #1689, #522, #8052, #6347, #10814, #4257, #3415, #10927, #2424, #4440, #763, #7300, #706, #10995, #1446, #6164, #2612, #8172, #4319, #11901, #9149, #4384, #11962, #2667, #7983, #10006, #5370, #3528, #10069, #11052, #8238, #5181, #6398, #2545, #8971, #9892, #9096, #10874, #11787, #11720, #1503, #7123, #650, #1564, #7242, #5238, #3344, #7061, #2485, #6219, #9946, #5303, #9037, #11843, #3472, #7181, #1742, #1021, #832, #10192, #7496, #9215, #7554, #4629, #5733, #10371, #1993, #8360, #2853, #892, #1928, #9460, #9335, #5664, #12082, #1809, #10255, #951, #26, #11241, #1077, #6522, #4569, #4808, #3648, #11109, #3887, #11179, #8491, #6634, #8299, #5548, #4688, #2912, #9395, #1867, #12023, #11295, #5478, #5604, #8547, #4753, #88, #3706, #3834, #142, #7429, #8426, #2792, #2727, #6576, #7609, #11353, #2977, #10124, #7365, #6458, #10309, #9277, #3774, #6874, #5908, #10551, #9638, #10435, #3094, #6697, #1259, #11419, #6813, #5791, #1133, #10616, #4867, #2054, #7736, #4990, #5850, #9516, #8605, #202, #270, #8727, #8669, #329, #3953, #2168, #4068, #4012, #1191, #7798, #2110, #7679, #3039, #6757, #4931, #11533, #10494, #11474, #3156, #9578, #7134, #4453, #2624, #4271, #6176, #663, #11010, #10019, #6232, #5193, #10079, #5319, #10885, #3485, #9903, #3604, #4331, #9108, #6356, #8986, #9960, #3427, #10827 ),
 .UNSPECIFIED., .F., .F.,
 ( 4, 2, 2, 2, 2, 2, 2, 2, 2, 2, 2, 2, 2, 2, 2, 2, 2, 2, 2, 2, 2, 2, 2, 2, 2, 2, 2, 2, 2, 2, 2, 2, 2, 2, 2, 2, 2, 2, 2, 2, 2, 2, 2, 2, 2, 2, 2, 2, 2, 2, 2, 2, 2, 2, 2, 2, 2, 2, 2, 2, 2, 2, 2, 2, 2, 2, 2, 2, 2, 2, 2, 2, 2, 2, 2, 2, 2, 2, 2, 2, 2, 2, 2, 2, 2, 2, 2, 2, 2, 2, 2, 2, 2, 2, 2, 2, 2, 2, 2, 2, 2, 2, 2, 4 ),
 ( 0.000000000000000000, 0.007812500000000000000, 0.01562500000000000000, 0.02343750000000000000, 0.03125000000000000000, 0.03906250000000000000, 0.04687500000000000000, 0.05468750000000000000, 0.06250000000000000000, 0.07031250000000000000, 0.07812500000000000000, 0.08593750000000000000, 0.09375000000000000000, 0.1015624999999999861, 0.1093750000000000000, 0.1171875000000000000, 0.1250000000000000000, 0.1328125000000000000, 0.1406250000000000000, 0.1484375000000000000, 0.1562500000000000000, 0.1640624999999999722, 0.1718750000000000000, 0.1796875000000000000, 0.1875000000000000000, 0.1953125000000000000, 0.2031249999999999722, 0.2109375000000000000, 0.2187500000000000000, 0.2265625000000000000, 0.2343750000000000000, 0.2421875000000000000, 0.2500000000000000000, 0.2578125000000000000, 0.2656250000000000000, 0.2734375000000000000, 0.2812500000000000000, 0.2890625000000000000, 0.2968750000000000000, 0.3046875000000000000, 0.3125000000000000000, 0.3203125000000000000, 0.3281249999999999445, 0.3359375000000000000, 0.3437500000000000000, 0.3515625000000000000, 0.3593750000000000000, 0.3671874999999999445, 0.3750000000000000000, 0.3828125000000000000, 0.3906250000000000000, 0.3984375000000000000, 0.4062499999999999445, 0.4140625000000000000, 0.4218750000000000000, 0.4296875000000000000, 0.4375000000000000000, 0.4453125000000000000, 0.4531250000000000000, 0.4609375000000000000, 0.4687500000000000000, 0.4765625000000000000, 0.4843750000000000000, 0.4921875000000000000, 0.5000000000000000000, 0.5078125000000000000, 0.5156250000000000000, 0.5234375000000000000, 0.5312500000000000000, 0.5390625000000000000, 0.5468750000000000000, 0.5546875000000000000, 0.5625000000000000000, 0.5703125000000000000, 0.5781250000000000000, 0.5859375000000000000, 0.5937500000000000000, 0.6015625000000000000, 0.6093750000000000000, 0.6171874999999998890, 0.6250000000000000000, 0.6328125000000000000, 0.6406250000000000000, 0.6484375000000000000, 0.6562499999999998890, 0.6640625000000000000, 0.6718750000000000000, 0.6796875000000000000, 0.6875000000000000000, 0.6953124999999998890, 0.7031250000000000000, 0.7109375000000000000, 0.7187500000000000000, 0.7265625000000000000, 0.7343749999999998890, 0.7421875000000000000, 0.7500000000000000000, 0.7656250000000000000, 0.7812500000000000000, 0.7968750000000000000, 0.8124999999999998890, 0.8281250000000000000, 0.8437500000000000000, 0.8499999999999999778 ),
 .UNSPECIFIED. ) ;
#1508=CARTESIAN_POINT ( 'NONE',  ( -5.862605222286285667, -1.923479314576677535, 3.747395293195558847E-16 ) ) ;
#1515=CARTESIAN_POINT ( 'NONE',  ( 5.343773788080183884, 10.82393792025544421, 10.00000000000000000 ) ) ;
#1525=CARTESIAN_POINT ( 'NONE',  ( 2.578468386369129117, 11.91291369680096857, 6.857782953271941950E-17 ) ) ;
#1531=CARTESIAN_POINT ( 'NONE',  ( 3.656769781543558917, 7.172433557890307121, 10.00000000000000000 ) ) ;
#1539=CARTESIAN_POINT ( 'NONE',  ( -5.125696908148163367, -9.212757455310160992, 10.00000000000000000 ) ) ;
#1542=CARTESIAN_POINT ( 'NONE',  ( 3.885483365683944257, 13.62125166200964976, 3.747395293195558847E-16 ) ) ;
#1551=DIRECTION ( 'NONE',  ( 0.000000000000000000, 0.000000000000000000, 1.000000000000000000 ) ) ;
#1555=CARTESIAN_POINT ( 'NONE',  ( -6.829322889802586616, -2.192323464439263514, 10.00000000000000000 ) ) ;
#1557=CARTESIAN_POINT ( 'NONE',  ( -8.209791827104812256, -6.297951179201748850, 6.857782953271941950E-17 ) ) ;
#1562=VERTEX_POINT ( 'NONE', #4497 ) ;
#1564=CARTESIAN_POINT ( 'NONE',  ( -4.054747718262374789, -11.96785467447666029, 10.00000000000000000 ) ) ;
#1569=CARTESIAN_POINT ( 'NONE',  ( -5.704017324792769905, 1.489539271746818772, 3.747395293195558847E-16 ) ) ;
#1591=CARTESIAN_POINT ( 'NONE',  ( 11.51680056346191883, -0.3781118375584790470, 6.857782953271941950E-17 ) ) ;
#1600=CARTESIAN_POINT ( 'NONE',  ( -6.925491926712309620, 5.292860106065908177, 10.00000000000000000 ) ) ;
#1608=CARTESIAN_POINT ( 'NONE',  ( 2.798030692817974341, 8.692477993603725750, 10.00000000000000000 ) ) ;
#1617=CARTESIAN_POINT ( 'NONE',  ( 4.212679447664376298, 6.814025269448777955, 3.747395293195558847E-16 ) ) ;
#1624=CARTESIAN_POINT ( 'NONE',  ( 5.312937634500610073, -1.259815497212794400, 10.00000000000000000 ) ) ;
#1626=CARTESIAN_POINT ( 'NONE',  ( 10.96671743108978525, -3.132869264233209439, 6.857782953271941950E-17 ) ) ;
#1631=EDGE_LOOP ( 'NONE', ( #9715, #6175, #6162, #10993 ) ) ;
#1632=CARTESIAN_POINT ( 'NONE',  ( -7.115032382426030644, -13.85544350050026807, 10.00000000000000000 ) ) ;
#1636=CARTESIAN_POINT ( 'NONE',  ( -1.784247137544765716, 5.123456263349895679, 3.747395293195558847E-16 ) ) ;
#1653=CARTESIAN_POINT ( 'NONE',  ( -2.061894914253512123, 6.087690860853031793, 6.857782953271941950E-17 ) ) ;
#1659=CARTESIAN_POINT ( 'NONE',  ( -4.491015865170432164, 3.510096388331073403, 10.00000000000000000 ) ) ;
#1665=CARTESIAN_POINT ( 'NONE',  ( 3.913389251769919586, -3.458713887698555922, 10.00000000000000000 ) ) ;
#1672=CARTESIAN_POINT ( 'NONE',  ( 1.445324715877976729, -3.701599742324197084, 3.747395293195558847E-16 ) ) ;
#1674=CARTESIAN_POINT ( 'NONE',  ( 0.000000000000000000, 0.000000000000000000, 0.000000000000000000 ) ) ;
#1679=CARTESIAN_POINT ( 'NONE',  ( -1.032305814202113092, 6.265050879046242471, 10.00000000000000000 ) ) ;
#1681=CARTESIAN_POINT ( 'NONE',  ( -7.040021908109678428, -0.4595208068204874041, 6.857782953271941950E-17 ) ) ;
#1689=CARTESIAN_POINT ( 'NONE',  ( -14.60057116351880069, -4.165219547604622541, 10.00000000000000000 ) ) ;
#1692=CARTESIAN_POINT ( 'NONE',  ( -1.790740696106538632, -6.394195405909704810, 3.747395293195558847E-16 ) ) ;
#1711=CARTESIAN_POINT ( 'NONE',  ( 7.402789038520873000, -0.9464297003978345835, 10.00000000000000000 ) ) ;
#1718=CARTESIAN_POINT ( 'NONE',  ( 4.382127860174850120, -16.35473703246190524, 6.857782953271941950E-17 ) ) ;
#1725=CARTESIAN_POINT ( 'NONE',  ( 7.357672848543031385, 2.125097602832226151, 3.747395293195558847E-16 ) ) ;
#1733=CARTESIAN_POINT ( 'NONE',  ( -3.542987847618818353, 5.503081486278154522, 6.857782953271941950E-17 ) ) ;
#1742=CARTESIAN_POINT ( 'NONE',  ( -11.32214898804313208, 3.633524203737720448, 10.00000000000000000 ) ) ;
#1746=CARTESIAN_POINT ( 'NONE',  ( -0.3758430365714711674, 11.29677535215814110, 3.747395293195558847E-16 ) ) ;
#1763=CARTESIAN_POINT ( 'NONE',  ( -12.61273389267802436, -8.731886703669292871, 3.747395293195558847E-16 ) ) ;
#1764=CARTESIAN_POINT ( 'NONE',  ( 6.242895496888662521, -5.302832405932363713, 6.857782953271941950E-17 ) ) ;
#1773=CARTESIAN_POINT ( 'NONE',  ( -6.036922680726761747, -0.4347383792561346771, 10.00000000000000000 ) ) ;
#1779=CARTESIAN_POINT ( 'NONE',  ( 0.0002901587068752367257, -4.749354241797645315, 10.00000000000000000 ) ) ;
#1790=CARTESIAN_POINT ( 'NONE',  ( 4.623190192904133689, -5.402202315098909580, 3.747395293195558847E-16 ) ) ;
#1796=CARTESIAN_POINT ( 'NONE',  ( 16.47843063274657993, -5.593696103119286001, 10.00000000000000000 ) ) ;
#1798=CARTESIAN_POINT ( 'NONE',  ( 8.527474615971319949, 0.9793716136081375145, 6.857782953271941950E-17 ) ) ;
#1809=CARTESIAN_POINT ( 'NONE',  ( 9.640149279600557009, 4.768118462334745011, 10.00000000000000000 ) ) ;
#1814=CARTESIAN_POINT ( 'NONE',  ( -7.370305768634978882, 4.727533884956530486, 3.747395293195558847E-16 ) ) ;
#1830=CARTESIAN_POINT ( 'NONE',  ( 13.24268851590353790, -2.403973981684889072, 3.747395293195558847E-16 ) ) ;
#1831=CARTESIAN_POINT ( 'NONE',  ( 5.312937634499088624, -1.259815497212412261, 6.857782953271941950E-17 ) ) ;
#1841=CARTESIAN_POINT ( 'NONE',  ( 3.571029491936648093, 3.388293644658559423, 10.00000000000000000 ) ) ;
#1845=DIRECTION ( 'NONE',  ( 0.000000000000000000, 0.000000000000000000, -1.000000000000000000 ) ) ;
#1846=CARTESIAN_POINT ( 'NONE',  ( -2.682496113117368797, -7.114254743909099510, 10.00000000000000000 ) ) ;
#1855=CARTESIAN_POINT ( 'NONE',  ( 4.140589500486089314, -5.731468560950439439, 3.747395293195558847E-16 ) ) ;
#1861=CARTESIAN_POINT ( 'NONE',  ( 4.698850784960272087, -6.565226861933591174, 6.857782953271941950E-17 ) ) ;
#1867=CARTESIAN_POINT ( 'NONE',  ( -3.937910939466569005, -8.732312745279401156, 10.00000000000000000 ) ) ;
#1875=CARTESIAN_POINT ( 'NONE',  ( 6.685168693379560878, -7.607270790100919555, 3.747395293195558847E-16 ) ) ;
#1889=CARTESIAN_POINT ( 'NONE',  ( 11.62709622633471618, -6.461356448465071622, 3.747395293195558847E-16 ) ) ;
#1890=CARTESIAN_POINT ( 'NONE',  ( -2.100379401128184664, -7.348625593045285065, 6.857782953271941950E-17 ) ) ;
#1905=CARTESIAN_POINT ( 'NONE',  ( -6.829322889802586616, -2.192323464439263514, 10.00000000000000000 ) ) ;
#1913=CARTESIAN_POINT ( 'NONE',  ( -13.83044629298881389, 5.462350471645223138, 10.00000000000000000 ) ) ;
#1919=CARTESIAN_POINT ( 'NONE',  ( -3.791520748785662587, -16.26028641251513207, 10.00000000000000000 ) ) ;
#1920=CARTESIAN_POINT ( 'NONE',  ( -5.542557460684657045, -4.854674288179716690, 6.857782953271941950E-17 ) ) ;
#1928=CARTESIAN_POINT ( 'NONE',  ( 4.889075487038677004, 9.929493272051477248, 10.00000000000000000 ) ) ;
#1930=CARTESIAN_POINT ( 'NONE',  ( -5.773631947676829412, 9.989728373610901713, 3.747395293195558847E-16 ) ) ;
#1933=CARTESIAN_POINT ( 'NONE',  ( 3.571029491936644540, 3.388293644658557646, 3.747395293195558847E-16 ) ) ;
#1947=CARTESIAN_POINT ( 'NONE',  ( 5.172292865810426576, -11.91455349003027564, 3.747395293195558847E-16 ) ) ;
#1954=CARTESIAN_POINT ( 'NONE',  ( -7.575117642440520882, -14.74712341115847103, 10.00000000000000000 ) ) ;
#1963=CARTESIAN_POINT ( 'NONE',  ( 14.22875512193218661, -2.589574901423981057, 6.857782953271941950E-17 ) ) ;
#1973=CARTESIAN_POINT ( 'NONE',  ( -8.499083411061075566, 11.86528080735166490, 10.00000000000000000 ) ) ;
#1993=CARTESIAN_POINT ( 'NONE',  ( -0.3758430365714709454, 11.29677535215814466, 10.00000000000000000 ) ) ;
#1996=CARTESIAN_POINT ( 'NONE',  ( 7.316052646047088714, -7.060001943526879487, 3.747395293195558847E-16 ) ) ;
#1997=CARTESIAN_POINT ( 'NONE',  ( -12.59589084681760518, 2.937805917057593863, 6.857782953271941950E-17 ) ) ;
#2009=CARTESIAN_POINT ( 'NONE',  ( -13.29946171776798280, 6.562258890817371793, 3.747395293195558847E-16 ) ) ;
#2027=CARTESIAN_POINT ( 'NONE',  ( -15.85416723795448846, 2.087521067385502693, 6.857782953271941950E-17 ) ) ;
#2035=CARTESIAN_POINT ( 'NONE',  ( 2.839002905302877799, -15.63284973865751049, 10.00000000000000000 ) ) ;
#2039=CARTESIAN_POINT ( 'NONE',  ( 16.47843063274904196, -5.593696103119284224, 6.857782953271941950E-17 ) ) ;
#2044=CARTESIAN_POINT ( 'NONE',  ( 5.564773995946421969, -12.83798980516408683, 10.00000000000000000 ) ) ;
#2054=CARTESIAN_POINT ( 'NONE',  ( 6.563569809674243416, -3.208372544468512721, 10.00000000000000000 ) ) ;
#2056=CARTESIAN_POINT ( 'NONE',  ( -7.130211940009574256, -7.605417807865423541, 10.00000000000000000 ) ) ;
#2057=CARTESIAN_POINT ( 'NONE',  ( 7.525577113297162946, 13.03378399180780534, 6.857782953271941950E-17 ) ) ;
#2067=CARTESIAN_POINT ( 'NONE',  ( 0.03696586647634135525, -4.250492970015754324, 2.216586794261376644E-16 ) ) ;
#2070=CARTESIAN_POINT ( 'NONE',  ( -5.008276813248563997, -11.55791719732261313, 3.747395293195558847E-16 ) ) ;
#2071=VECTOR ( 'NONE', #5339, 1000.000000000000000 ) ;
#2075=SHAPE_DEFINITION_REPRESENTATION ( #5024, #7555 ) ;
#2076=CARTESIAN_POINT ( 'NONE',  ( 0.2749788638910979355, -16.81181333738675931, 10.00000000000000000 ) ) ;
#2085=CARTESIAN_POINT ( 'NONE',  ( -12.59589084681760518, 2.937805917057593863, 6.857782953271941950E-17 ) ) ;
#2094=CARTESIAN_POINT ( 'NONE',  ( -1.036640877615905287, -15.73686152240404823, 10.00000000000000000 ) ) ;
#2099=CARTESIAN_POINT ( 'NONE',  ( -11.39998097177319636, 5.856612080558658562, 10.00000000000000000 ) ) ;
#2101=CARTESIAN_POINT ( 'NONE',  ( 0.4634152073531430105, 14.27464310366533340, 3.747395293195558847E-16 ) ) ;
#2110=CARTESIAN_POINT ( 'NONE',  ( -5.319913005755715574, -3.351504787099933047, 10.00000000000000000 ) ) ;
#2112=CARTESIAN_POINT ( 'NONE',  ( 8.393308867179015920, -1.106660293010312657, 10.00000000000000000 ) ) ;
#2113=CARTESIAN_POINT ( 'NONE',  ( 14.27634331491212016, 3.322769473268863738, 6.857782953271941950E-17 ) ) ;
#2124=CARTESIAN_POINT ( 'NONE',  ( 10.51453309316909213, -0.3307463982597989571, 3.747395293195558847E-16 ) ) ;
#2131=CARTESIAN_POINT ( 'NONE',  ( 11.73504485001147835, -12.52947377801879192, 10.00000000000000000 ) ) ;
#2143=CARTESIAN_POINT ( 'NONE',  ( -16.06046882360139350, -0.5196555361422402486, 6.857782953271941950E-17 ) ) ;
#2151=CARTESIAN_POINT ( 'NONE',  ( 5.172292865810427465, -11.91455349003027919, 10.00000000000000000 ) ) ;
#2158=CARTESIAN_POINT ( 'NONE',  ( -12.59589084681761229, 2.937805917057824789, 10.00000000000000000 ) ) ;
#2168=CARTESIAN_POINT ( 'NONE',  ( -2.296015608618633852, -6.188270089872266233, 10.00000000000000000 ) ) ;
#2173=CARTESIAN_POINT ( 'NONE',  ( -0.1814876354083667931, -10.77628937513455654, 10.00000000000000000 ) ) ;
#2174=CARTESIAN_POINT ( 'NONE',  ( 14.53830338343599848, -0.2437330612273620467, 6.857782953271941950E-17 ) ) ;
#2183=CARTESIAN_POINT ( 'NONE',  ( 15.52845182490561626, -5.270724383582042982, 10.00000000000000000 ) ) ;
#2189=CARTESIAN_POINT ( 'NONE',  ( -11.15100792855598755, -5.055838994807843711, 3.747395293195558847E-16 ) ) ;
#2196=CARTESIAN_POINT ( 'NONE',  ( 1.748316258820582947, 15.14524454193559144, 10.00000000000000000 ) ) ;
#2205=CARTESIAN_POINT ( 'NONE',  ( -12.91830213043053988, -2.344901317288421883, 6.857782953271941950E-17 ) ) ;
#2214=CARTESIAN_POINT ( 'NONE',  ( 7.078846155420733588, 8.354583459611244933, 10.00000000000000000 ) ) ;
#2222=CARTESIAN_POINT ( 'NONE',  ( 11.20109743375192224, 9.815261043520028039, 10.00000000000000000 ) ) ;
#2225=FACE_OUTER_BOUND ( 'NONE', #1631, .T. ) ;
#2234=CARTESIAN_POINT ( 'NONE',  ( 6.986659217179110648, 9.748146710219847577, 10.00000000000000000 ) ) ;
#2235=CARTESIAN_POINT ( 'NONE',  ( 8.588976300537435549, -11.19439025337200810, 6.857782953271941950E-17 ) ) ;
#2249=CARTESIAN_POINT ( 'NONE',  ( -5.868204859621548586, -7.421994279450896848, 3.747395293195558847E-16 ) ) ;
#2256=CARTESIAN_POINT ( 'NONE',  ( 13.14573027368779456, 6.745762002080610387, 10.00000000000000000 ) ) ;
#2259=CARTESIAN_POINT ( 'NONE',  ( 17.50000000000000000, 0.000000000000000000, 10.00000000000000000 ) ) ;
#2266=CARTESIAN_POINT ( 'NONE',  ( 11.40744677810890373, -1.317628706759688129, 6.857782953271941950E-17 ) ) ;
#2273=CARTESIAN_POINT ( 'NONE',  ( -0.1481022647113163504, -9.773457036294484368, 10.00000000000000000 ) ) ;
#2278=CARTESIAN_POINT ( 'NONE',  ( -10.84705874452746777, 6.751620637726422736, 10.00000000000000000 ) ) ;
#2291=CARTESIAN_POINT ( 'NONE',  ( 11.50231346626665996, 1.508968394323198847, 10.00000000000000000 ) ) ;
#2292=CARTESIAN_POINT ( 'NONE',  ( 1.597090680284417363, 12.12373805211590749, 6.857782953271941950E-17 ) ) ;
#2303=CARTESIAN_POINT ( 'NONE',  ( -12.04643853703213452, -0.2059847383342608973, 3.747395293195558847E-16 ) ) ;
#2309=CARTESIAN_POINT ( 'NONE',  ( 1.597090680284417807, 12.12373805211591460, 10.00000000000000000 ) ) ;
#2322=CARTESIAN_POINT ( 'NONE',  ( 7.334967666341834835, -8.371827447635054043, 6.857782953271941950E-17 ) ) ;
#2330=CARTESIAN_POINT ( 'NONE',  ( 2.257301671556971367, -9.631158585656901749, 10.00000000000000000 ) ) ;
#2338=CARTESIAN_POINT ( 'NONE',  ( 4.138106518799270717, 8.052838533163344081, 10.00000000000000000 ) ) ;
#2340=CARTESIAN_POINT ( 'NONE',  ( 13.53515989517831564, -0.2218654272304620700, 3.747395293195558847E-16 ) ) ;
#2345=CARTESIAN_POINT ( 'NONE',  ( 17.49999999999999645, 0.000000000000000000, 6.857782953271941950E-17 ) ) ;
#2350=CARTESIAN_POINT ( 'NONE',  ( -5.152979166089619589, -5.321787192520355703, 10.00000000000000000 ) ) ;
#2351=CARTESIAN_POINT ( 'NONE',  ( -4.389456771235329846, 11.66511648340389051, 6.857782953271941950E-17 ) ) ;
#2365=AXIS2_PLACEMENT_3D ( 'NONE', #990, #4732, #8468 ) ;
#2367=CARTESIAN_POINT ( 'NONE',  ( 2.467392210070199710, 7.745125807189173095, 3.747395293195558847E-16 ) ) ;
#2373=CARTESIAN_POINT ( 'NONE',  ( 2.578468386369561216, 11.91291369680097567, 10.00000000000000000 ) ) ;
#2383=CARTESIAN_POINT ( 'NONE',  ( 10.63538685525200478, -4.008487272325076844, 6.857782953271941950E-17 ) ) ;
#2391=CARTESIAN_POINT ( 'NONE',  ( -10.51222845931418703, 5.388985543801221745, 10.00000000000000000 ) ) ;
#2399=CARTESIAN_POINT ( 'NONE',  ( -2.764021070441486039, -10.29567250283336399, 10.00000000000000000 ) ) ;
#2401=CARTESIAN_POINT ( 'NONE',  ( -9.045553118584754415, -8.482981269326389295, 3.747395293195558847E-16 ) ) ;
#2414=CARTESIAN_POINT ( 'NONE',  ( -6.661525743073271499, 1.789546221321743458, 10.00000000000000000 ) ) ;
#2416=CARTESIAN_POINT ( 'NONE',  ( -0.3972327064967883237, 12.29993208790119930, 6.857782953271941950E-17 ) ) ;
#2424=CARTESIAN_POINT ( 'NONE',  ( -11.21689850596896676, 9.520844388990630236, 10.00000000000000000 ) ) ;
#2429=CARTESIAN_POINT ( 'NONE',  ( 6.563569809674826061, -3.208372544468511833, 3.747395293195558847E-16 ) ) ;
#2435=CARTESIAN_POINT ( 'NONE',  ( 13.92981926110968161, -3.738495919395732781, 10.00000000000000000 ) ) ;
#2445=CARTESIAN_POINT ( 'NONE',  ( 9.774996403550728630, -5.644905071530503804, 6.857782953271941950E-17 ) ) ;
#2450=CARTESIAN_POINT ( 'NONE',  ( 10.00611923916671309, -2.842981073525690405, 10.00000000000000000 ) ) ;
#2458=CARTESIAN_POINT ( 'NONE',  ( 8.025946968469186871, -7.769110617520879281, 10.00000000000000000 ) ) ;
#2460=CARTESIAN_POINT ( 'NONE',  ( 2.103398428914359020, -12.69820342197950680, 3.747395293195558847E-16 ) ) ;
#2468=B_SPLINE_CURVE_WITH_KNOTS ( 'NONE', 3,
 ( #10420, #5834, #7664, #2039, #4850, #5779, #8591, #8698, #11497, #3119, #5938, #6779, #281, #10504, #9653, #9451, #4801, #7613, #1313, #6704, #7803, #5854, #147, #3217, #8611, #7868, #6881, #6935, #334, #10439, #1080, #10624, #9643, #11422, #6761, #4137, #1198, #10497, #9584, #4813, #273, #6817, #5049, #2057, #2982, #3043, #5795, #4015, #8550, #11538, #2113, #4873, #2174, #3893, #8788, #4937, #9520, #8673, #11357, #2235, #1262, #4994, #5972, #10556, #11601, #5740, #4072, #1137, #7741, #11478, #9701, #3098, #7685, #5916, #208, #393, #3957, #8732, #3162, #1997, #9463, #10806, #9757, #2536, #9884, #3334, #8044, #2351, #8165, #4434, #2416, #2292, #2478, #9999, #456, #3406, #6157, #3270, #6211, #6273, #4309, #7175, #9936, #8852, #5108, #1626, #5361, #7115, #11778, #6028, #1439, #9825, #4195, #3466, #1376, #7922, #10918, #4376, #10867, #8109, #11893, #9090, #11836, #1557, #699, #10680, #11654, #1497, #6992, #10739, #5229, #3521, #6092, #5293, #5172, #9030, #8908, #641, #514, #11712, #4249, #7976, #7053, #8962, #575, #757, #8227, #943, #6512, #8291, #7357, #5415, #7294, #1798, #12, #11168, #11101, #6340, #11231, #6450, #12017, #8414, #1861, #5596, #5469, #10246, #3764, #11952, #9386, #2718, #3582, #12073, #7486, #8483, #1920, #9327, #2843, #2781, #9142, #1681, #6568, #7419, #4679, #1009, #5537, #6391, #10302, #2605, #1733, #5656, #4493, #10062, #9203, #4622, #3641, #10115, #4743, #79, #7233, #10986, #11047, #10182, #2660, #822, #9267, #4559, #886, #8354 ),
 .UNSPECIFIED., .F., .F.,
 ( 4, 2, 2, 2, 2, 2, 2, 2, 2, 2, 2, 2, 2, 2, 2, 2, 2, 2, 2, 2, 2, 2, 2, 2, 2, 2, 2, 2, 2, 2, 2, 2, 2, 2, 2, 2, 2, 2, 2, 2, 2, 2, 2, 2, 2, 2, 2, 2, 2, 2, 2, 2, 2, 2, 2, 2, 2, 2, 2, 2, 2, 2, 2, 2, 2, 2, 2, 2, 2, 2, 2, 2, 2, 2, 2, 2, 2, 2, 2, 2, 2, 2, 2, 2, 2, 2, 2, 2, 2, 2, 2, 2, 2, 2, 2, 2, 2, 2, 2, 2, 2, 2, 2, 4 ),
 ( 0.000000000000000000, 0.007812500000000000000, 0.01562500000000000000, 0.02343750000000000000, 0.03125000000000000000, 0.03906250000000000000, 0.04687500000000000000, 0.05468750000000000000, 0.06250000000000000000, 0.07031250000000000000, 0.07812500000000000000, 0.08593750000000000000, 0.09375000000000000000, 0.1015624999999999861, 0.1093750000000000000, 0.1171875000000000000, 0.1250000000000000000, 0.1328125000000000000, 0.1406250000000000000, 0.1484375000000000000, 0.1562500000000000000, 0.1640624999999999722, 0.1718750000000000000, 0.1796875000000000000, 0.1875000000000000000, 0.1953125000000000000, 0.2031249999999999722, 0.2109375000000000000, 0.2187500000000000000, 0.2265625000000000000, 0.2343750000000000000, 0.2421875000000000000, 0.2500000000000000000, 0.2578125000000000000, 0.2656250000000000000, 0.2734375000000000000, 0.2812500000000000000, 0.2890625000000000000, 0.2968750000000000000, 0.3046875000000000000, 0.3125000000000000000, 0.3203125000000000000, 0.3281249999999999445, 0.3359375000000000000, 0.3437500000000000000, 0.3515625000000000000, 0.3593750000000000000, 0.3671874999999999445, 0.3750000000000000000, 0.3828125000000000000, 0.3906250000000000000, 0.3984375000000000000, 0.4062499999999999445, 0.4140625000000000000, 0.4218750000000000000, 0.4296875000000000000, 0.4375000000000000000, 0.4453125000000000000, 0.4531250000000000000, 0.4609375000000000000, 0.4687500000000000000, 0.4765625000000000000, 0.4843750000000000000, 0.4921875000000000000, 0.5000000000000000000, 0.5078125000000000000, 0.5156250000000000000, 0.5234375000000000000, 0.5312500000000000000, 0.5390625000000000000, 0.5468750000000000000, 0.5546875000000000000, 0.5625000000000000000, 0.5703125000000000000, 0.5781250000000000000, 0.5859375000000000000, 0.5937500000000000000, 0.6015625000000000000, 0.6093750000000000000, 0.6171874999999998890, 0.6250000000000000000, 0.6328125000000000000, 0.6406250000000000000, 0.6484375000000000000, 0.6562499999999998890, 0.6640625000000000000, 0.6718750000000000000, 0.6796875000000000000, 0.6875000000000000000, 0.6953124999999998890, 0.7031250000000000000, 0.7109375000000000000, 0.7187500000000000000, 0.7265625000000000000, 0.7343749999999998890, 0.7421875000000000000, 0.7500000000000000000, 0.7656250000000000000, 0.7812500000000000000, 0.7968750000000000000, 0.8124999999999998890, 0.8281250000000000000, 0.8437500000000000000, 0.8499999999999999778 ),
 .UNSPECIFIED. ) ;
#2478=CARTESIAN_POINT ( 'NONE',  ( 2.578468386369129117, 11.91291369680096857, 6.857782953271941950E-17 ) ) ;
#2485=CARTESIAN_POINT ( 'NONE',  ( -9.680665087126289592, -7.686621967951973389, 10.00000000000000000 ) ) ;
#2488=CARTESIAN_POINT ( 'NONE',  ( -6.036922680726758195, -0.4347383792561972382, 3.747395293195558847E-16 ) ) ;
#2504=CARTESIAN_POINT ( 'NONE',  ( 2.084091085258986009, 8.931495281877380066, 6.857782953271941950E-17 ) ) ;
#2512=CARTESIAN_POINT ( 'NONE',  ( -6.012500708481080203, 0.06204199954272103523, 10.00000000000000000 ) ) ;
#2520=CARTESIAN_POINT ( 'NONE',  ( 6.396238541183701720, 6.183590428399974748, 10.00000000000000000 ) ) ;
#2528=CARTESIAN_POINT ( 'NONE',  ( 4.525508228541170297, -0.2388087992699348128, 3.747395293195558847E-16 ) ) ;
#2534=CARTESIAN_POINT ( 'NONE',  ( 0.3111040546027374343, -4.780743156735979049, 10.00000000000000000 ) ) ;
#2536=CARTESIAN_POINT ( 'NONE',  ( -9.546882484473291797, 8.373557015400844961, 6.857782953271941950E-17 ) ) ;
#2545=CARTESIAN_POINT ( 'NONE',  ( 10.36190401371066727, -8.216093097539268086, 10.00000000000000000 ) ) ;
#2551=CARTESIAN_POINT ( 'NONE',  ( 6.411932913580776550, 4.469049885107575726, 3.747395293195558847E-16 ) ) ;
#2570=CARTESIAN_POINT ( 'NONE',  ( 0.3111040546027372677, -4.780743156735971944, 6.857782953271941950E-17 ) ) ;
#2580=CARTESIAN_POINT ( 'NONE',  ( 7.527773320476329744, 0.8933511214756656438, 10.00000000000000000 ) ) ;
#2590=CARTESIAN_POINT ( 'NONE',  ( 8.235329212248927888, -1.783486464602662691, 10.00000000000000000 ) ) ;
#2597=CARTESIAN_POINT ( 'NONE',  ( -0.1881845630465192321, -6.755137126427047001, 3.747395293195558847E-16 ) ) ;
#2600=ORIENTED_EDGE ( 'NONE', *, *, #4533, .T. ) ;
#2603=CARTESIAN_POINT ( 'NONE',  ( -0.8869411547437835441, -7.669649013129178350, 10.00000000000000000 ) ) ;
#2605=CARTESIAN_POINT ( 'NONE',  ( -4.006926059188537614, 5.225193401749451461, 6.857782953271941950E-17 ) ) ;
#2612=CARTESIAN_POINT ( 'NONE',  ( 1.629745903656676820, 14.14889381255350287, 10.00000000000000000 ) ) ;
#2615=CARTESIAN_POINT ( 'NONE',  ( 7.357672848543031385, 2.125097602832226151, 3.747395293195558847E-16 ) ) ;
#2624=CARTESIAN_POINT ( 'NONE',  ( -3.432991321284830200, 4.402131891631372973, 10.00000000000000000 ) ) ;
#2629=CARTESIAN_POINT ( 'NONE',  ( -5.542557460684657045, -4.854674288179716690, 6.857782953271941950E-17 ) ) ;
#2633=ORIENTED_EDGE ( 'NONE', *, *, #7856, .F. ) ;
#2637=CARTESIAN_POINT ( 'NONE',  ( -7.370305768634982435, 4.727533884956532262, 10.00000000000000000 ) ) ;
#2644=CARTESIAN_POINT ( 'NONE',  ( 8.281812197879517612, -14.90260015151217488, 6.857782953271941950E-17 ) ) ;
#2650=VECTOR ( 'NONE', #10799, 1000.000000000000000 ) ;
#2651=CARTESIAN_POINT ( 'NONE',  ( 3.120778274233606098, -6.257845451233481349, 3.747395293195558847E-16 ) ) ;
#2653=DIRECTION ( 'NONE',  ( 1.000000000000000000, 0.000000000000000000, 0.000000000000000000 ) ) ;
#2657=CARTESIAN_POINT ( 'NONE',  ( -15.18624859168667918, -5.715447929355455869, 10.00000000000000000 ) ) ;
#2660=CARTESIAN_POINT ( 'NONE',  ( 3.913389251770639010, -3.458713887698550593, 6.857782953271941950E-17 ) ) ;
#2667=CARTESIAN_POINT ( 'NONE',  ( 11.72652038055310086, 7.297668919378235586, 10.00000000000000000 ) ) ;
#2670=CARTESIAN_POINT ( 'NONE',  ( 2.467392210070199710, 7.745125807189173095, 3.747395293195558847E-16 ) ) ;
#2671=CARTESIAN_POINT ( 'NONE',  ( 1.445324715877976729, -3.701599742324197084, 3.747395293195558847E-16 ) ) ;
#2684=CARTESIAN_POINT ( 'NONE',  ( -2.682496113117365244, -7.114254743909630641, 6.857782953271941950E-17 ) ) ;
#2692=CARTESIAN_POINT ( 'NONE',  ( -5.315861670734006061, 2.363279591656077816, 10.00000000000000000 ) ) ;
#2701=CARTESIAN_POINT ( 'NONE',  ( -6.947552178111049415, -1.615339808524829168, 10.00000000000000000 ) ) ;
#2708=CARTESIAN_POINT ( 'NONE',  ( -5.862605222286285667, -1.923479314576677535, 3.747395293195558847E-16 ) ) ;
#2718=CARTESIAN_POINT ( 'NONE',  ( -2.100379401128184664, -7.348625593045285065, 6.857782953271941950E-17 ) ) ;
#2727=CARTESIAN_POINT ( 'NONE',  ( -7.370305768634982435, 4.727533884956532262, 10.00000000000000000 ) ) ;
#2733=CARTESIAN_POINT ( 'NONE',  ( 8.282588618525734248, 7.043362411858246297, 3.747395293195558847E-16 ) ) ;
#2735=CARTESIAN_POINT ( 'NONE',  ( 4.321204520403003180, 2.017656881711011430, 3.747395293195558847E-16 ) ) ;
#2746=CARTESIAN_POINT ( 'NONE',  ( -11.08238827499517321, -10.71925978067678642, 3.747395293195558847E-16 ) ) ;
#2747=CARTESIAN_POINT ( 'NONE',  ( -5.924299593718516554, 3.297400215539475710, 6.857782953271941950E-17 ) ) ;
#2755=CARTESIAN_POINT ( 'NONE',  ( -2.214925388402925410, 4.996014981202114846, 10.00000000000000000 ) ) ;
#2757=DIRECTION ( 'NONE',  ( -0.000000000000000000, 1.000000000000000000, 0.000000000000000000 ) ) ;
#2762=CARTESIAN_POINT ( 'NONE',  ( 15.92723891616420673, -6.911623607273379655, 6.857782953271941950E-17 ) ) ;
#2774=CARTESIAN_POINT ( 'NONE',  ( -0.4771094043438768861, 5.286185534804329400, 3.747395293195558847E-16 ) ) ;
#2780=CARTESIAN_POINT ( 'NONE',  ( 8.281812197879521165, -14.90260015151097228, 10.00000000000000000 ) ) ;
#2781=CARTESIAN_POINT ( 'NONE',  ( -6.829322889802579510, -2.192323464439260849, 6.857782953271941950E-17 ) ) ;
#2792=CARTESIAN_POINT ( 'NONE',  ( -8.111627617515260624, 3.498804908652024093, 10.00000000000000000 ) ) ;
#2797=CARTESIAN_POINT ( 'NONE',  ( 2.257301671556970479, -9.631158585656898197, 3.747395293195558847E-16 ) ) ;
#2815=CARTESIAN_POINT ( 'NONE',  ( 4.977139221860116258, 13.21892491369776934, 3.747395293195558847E-16 ) ) ;
#2816=CARTESIAN_POINT ( 'NONE',  ( 2.529667540516381319, -4.392173529266732324, 6.857782953271941950E-17 ) ) ;
#2830=CARTESIAN_POINT ( 'NONE',  ( -2.100379401128186441, -7.348625593045292170, 10.00000000000000000 ) ) ;
#2838=CARTESIAN_POINT ( 'NONE',  ( -9.470608727121586412, 11.15741021143934653, 10.00000000000000000 ) ) ;
#2842=CARTESIAN_POINT ( 'NONE',  ( -15.59049818040342927, 3.373450308083567606, 10.00000000000000000 ) ) ;
#2843=CARTESIAN_POINT ( 'NONE',  ( -6.451445390047170214, -3.308750875808896819, 6.857782953271941950E-17 ) ) ;
#2853=CARTESIAN_POINT ( 'NONE',  ( 2.355103038863951781, 10.93470652055904146, 10.00000000000000000 ) ) ;
#2858=CARTESIAN_POINT ( 'NONE',  ( -3.516813791735896810, 7.717845097288992484, 3.747395293195558847E-16 ) ) ;
#2872=CARTESIAN_POINT ( 'NONE',  ( -13.25288834650809555, -7.646628085888695914, 3.747395293195558847E-16 ) ) ;
#2886=CARTESIAN_POINT ( 'NONE',  ( 11.20109743375191691, 9.815261043521076090, 6.857782953271941950E-17 ) ) ;
#2896=CARTESIAN_POINT ( 'NONE',  ( -10.19073739998278683, -11.62312336453203798, 10.00000000000000000 ) ) ;
#2902=CARTESIAN_POINT ( 'NONE',  ( 1.748316258820582947, 15.14524454193559144, 10.00000000000000000 ) ) ;
#2912=CARTESIAN_POINT ( 'NONE',  ( -1.719633853164447057, -9.543036404944420070, 10.00000000000000000 ) ) ;
#2914=CARTESIAN_POINT ( 'NONE',  ( 10.51453309316909213, -0.3307463982597989571, 3.747395293195558847E-16 ) ) ;
#2933=CARTESIAN_POINT ( 'NONE',  ( 2.103398428914359020, -12.69820342197950680, 3.747395293195558847E-16 ) ) ;
#2942=DIRECTION ( 'NONE',  ( 0.000000000000000000, -0.000000000000000000, 1.000000000000000000 ) ) ;
#2948=CARTESIAN_POINT ( 'NONE',  ( 14.53830338343599848, -0.2437330612273620467, 6.857782953271941950E-17 ) ) ;
#2953=ORIENTED_EDGE ( 'NONE', *, *, #4211, .F. ) ;
#2960=CARTESIAN_POINT ( 'NONE',  ( 13.68367311611256909, -8.822018488634764566, 10.00000000000000000 ) ) ;
#2967=CARTESIAN_POINT ( 'NONE',  ( -11.61414229320030778, -6.453515506896109422, 10.00000000000000000 ) ) ;
#2977=CARTESIAN_POINT ( 'NONE',  ( -4.158289900078591117, 7.437556212722741478, 10.00000000000000000 ) ) ;
#2980=CARTESIAN_POINT ( 'NONE',  ( -9.820986981723351050, 1.626514086989862662, 10.00000000000000000 ) ) ;
#2982=CARTESIAN_POINT ( 'NONE',  ( 8.547432504762587868, 12.33942397201039753, 6.857782953271941950E-17 ) ) ;
#2994=CARTESIAN_POINT ( 'NONE',  ( 9.683839015878911383, 10.01260560230520547, 3.747395293195558847E-16 ) ) ;
#3002=CARTESIAN_POINT ( 'NONE',  ( 3.017784444055084947, -16.62017357425736463, 10.00000000000000000 ) ) ;
#3012=FACE_OUTER_BOUND ( 'NONE', #4439, .T. ) ;
#3013=CARTESIAN_POINT ( 'NONE',  ( -1.124919223378054722, -13.71093750358708085, 6.857782953271941950E-17 ) ) ;
#3023=CARTESIAN_POINT ( 'NONE',  ( 12.25096627321952170, 6.291700371256734314, 10.00000000000000000 ) ) ;
#3029=CARTESIAN_POINT ( 'NONE',  ( 8.588976300537440878, -11.19439025337201343, 10.00000000000000000 ) ) ;
#3031=CARTESIAN_POINT ( 'NONE',  ( -8.499083411061073789, 11.86528080735276269, 3.747395293195558847E-16 ) ) ;
#3039=CARTESIAN_POINT ( 'NONE',  ( -5.862605222286289219, -1.923479314576678423, 10.00000000000000000 ) ) ;
#3042=CARTESIAN_POINT ( 'NONE',  ( 4.764169229607557732, 7.652272242165495619, 10.00000000000000000 ) ) ;
#3043=CARTESIAN_POINT ( 'NONE',  ( 10.38524206949620243, 10.73010674553377264, 6.857782953271941950E-17 ) ) ;
#3053=CARTESIAN_POINT ( 'NONE',  ( 7.078846155421574693, 8.354583459611243157, 3.747395293195558847E-16 ) ) ;
#3069=CARTESIAN_POINT ( 'NONE',  ( -9.783806739528728258, -9.162509837619118969, 6.857782953271941950E-17 ) ) ;
#3078=CARTESIAN_POINT ( 'NONE',  ( 10.36190401371066727, -8.216093097539268086, 10.00000000000000000 ) ) ;
#3085=CARTESIAN_POINT ( 'NONE',  ( 11.40744677810891083, -1.317628706759891966, 10.00000000000000000 ) ) ;
#3087=CARTESIAN_POINT ( 'NONE',  ( -12.61273389267802436, -8.731886703669292871, 3.747395293195558847E-16 ) ) ;
#3094=CARTESIAN_POINT ( 'NONE',  ( 6.411932913581408044, 4.469049885107577502, 10.00000000000000000 ) ) ;
#3097=CARTESIAN_POINT ( 'NONE',  ( 9.774996403550735735, -5.644905071530105900, 10.00000000000000000 ) ) ;
#3098=CARTESIAN_POINT ( 'NONE',  ( -9.783806739528728258, -9.162509837619118969, 6.857782953271941950E-17 ) ) ;
#3107=CARTESIAN_POINT ( 'NONE',  ( 15.00667705184754119, -6.512453894250635145, 10.00000000000000000 ) ) ;
#3113=CARTESIAN_POINT ( 'NONE',  ( -11.62103867303406624, 2.700230667072888835, 3.747395293195558847E-16 ) ) ;
#3117=CARTESIAN_POINT ( 'NONE',  ( 13.67726327739690184, -10.50289975150004018, 10.00000000000000000 ) ) ;
#3119=CARTESIAN_POINT ( 'NONE',  ( 8.281812197879517612, -14.90260015151217488, 6.857782953271941950E-17 ) ) ;
#3128=CARTESIAN_POINT ( 'NONE',  ( -12.06849956494802889, -5.462025159506374017, 6.857782953271941950E-17 ) ) ;
#3134=CARTESIAN_POINT ( 'NONE',  ( 8.429646098664189680, -5.822225404888640377, 10.00000000000000000 ) ) ;
#3138=CARTESIAN_POINT ( 'NONE',  ( 13.99323099383125069, 4.495563823643928814, 10.00000000000000000 ) ) ;
#3156=CARTESIAN_POINT ( 'NONE',  ( -5.315861670734006061, 2.363279591656077816, 10.00000000000000000 ) ) ;
#3160=CARTESIAN_POINT ( 'NONE',  ( -1.916691774771272172, -10.52688368019216725, 10.00000000000000000 ) ) ;
#3162=CARTESIAN_POINT ( 'NONE',  ( -12.98359546555289334, 0.8565524458115012507, 6.857782953271941950E-17 ) ) ;
#3170=CARTESIAN_POINT ( 'NONE',  ( 10.01890055165175042, -12.63311126014650121, 10.00000000000000000 ) ) ;
#3175=CARTESIAN_POINT ( 'NONE',  ( -8.694522232909450921, -2.966707450564700199, 3.747395293195558847E-16 ) ) ;
#3181=CARTESIAN_POINT ( 'NONE',  ( -2.240087900411203758, -13.53314956822678639, 10.00000000000000000 ) ) ;
#3191=CARTESIAN_POINT ( 'NONE',  ( 11.37845468071831512, 2.456417158213069829, 6.857782953271941950E-17 ) ) ;
#3200=CARTESIAN_POINT ( 'NONE',  ( 4.889075487038677004, 9.929493272051477248, 10.00000000000000000 ) ) ;
#3204=CARTESIAN_POINT ( 'NONE',  ( 8.547432504761534489, 12.33942397201040286, 10.00000000000000000 ) ) ;
#3216=CARTESIAN_POINT ( 'NONE',  ( 0.6097887191948987429, 9.229167205757272896, 10.00000000000000000 ) ) ;
#3217=CARTESIAN_POINT ( 'NONE',  ( -15.18624859168667562, -5.715447929355453205, 6.857782953271941950E-17 ) ) ;
#3228=CARTESIAN_POINT ( 'NONE',  ( 8.282588618525734248, 7.043362411858246297, 3.747395293195558847E-16 ) ) ;
#3233=CARTESIAN_POINT ( 'NONE',  ( 14.54887842078032989, 0.9530482589066729959, 10.00000000000000000 ) ) ;
#3242=CARTESIAN_POINT ( 'NONE',  ( -0.3972327064967883237, 12.29993208790119930, 6.857782953271941950E-17 ) ) ;
#3250=CARTESIAN_POINT ( 'NONE',  ( -8.962830026514758686, 0.7152994853347287574, 10.00000000000000000 ) ) ;
#3258=CARTESIAN_POINT ( 'NONE',  ( -4.625218816435448410, 8.325684435358759572, 10.00000000000000000 ) ) ;
#3261=CARTESIAN_POINT ( 'NONE',  ( -5.008276813248563997, -11.55791719732261313, 3.747395293195558847E-16 ) ) ;
#3269=CARTESIAN_POINT ( 'NONE',  ( -6.947552178111049415, -1.615339808524829168, 10.00000000000000000 ) ) ;
#3270=CARTESIAN_POINT ( 'NONE',  ( 9.056240860197961595, 7.682302481599242228, 6.857782953271941950E-17 ) ) ;
#3277=CARTESIAN_POINT ( 'NONE',  ( -1.036640877615905287, -15.73686152240404823, 10.00000000000000000 ) ) ;
#3282=CARTESIAN_POINT ( 'NONE',  ( 5.319643049700911952, -8.526005966358411570, 3.747395293195558847E-16 ) ) ;
#3288=CARTESIAN_POINT ( 'NONE',  ( -6.266017822847497420, 10.86399168115691438, 10.00000000000000000 ) ) ;
#3294=PRODUCT_DEFINITION_CONTEXT ( 'detailed design', #6150, 'design' ) ;
#3299=CARTESIAN_POINT ( 'NONE',  ( 4.138106518798946531, 8.052838533163340529, 6.857782953271941950E-17 ) ) ;
#3306=CARTESIAN_POINT ( 'NONE',  ( -8.109405675831295568, 8.372220220303479010, 10.00000000000000000 ) ) ;
#3316=CARTESIAN_POINT ( 'NONE',  ( 1.018538006779725835, -7.771884277300785904, 10.00000000000000000 ) ) ;
#3320=CARTESIAN_POINT ( 'NONE',  ( -11.98301361336074145, 0.7816210414391653316, 3.747395293195558847E-16 ) ) ;
#3334=CARTESIAN_POINT ( 'NONE',  ( -7.159234172427924925, 10.34564589702410942, 6.857782953271941950E-17 ) ) ;
#3344=CARTESIAN_POINT ( 'NONE',  ( -7.594692469639083399, -9.901549393538205734, 10.00000000000000000 ) ) ;
#3350=CARTESIAN_POINT ( 'NONE',  ( -8.834572391846261752, 1.442725564903823532, 3.747395293195558847E-16 ) ) ;
#3357=CARTESIAN_POINT ( 'NONE',  ( -12.91830213043054698, -2.344901317288422327, 10.00000000000000000 ) ) ;
#3362=DIRECTION ( 'NONE',  ( -2.303929616531696922E-17, 1.860490927985125609E-14, 1.000000000000000000 ) ) ;
#3370=CARTESIAN_POINT ( 'NONE',  ( 5.835571643920552276, -9.386589068694823013, 6.857782953271941950E-17 ) ) ;
#3376=CARTESIAN_POINT ( 'NONE',  ( -11.62103867303406979, 2.700230667072889279, 10.00000000000000000 ) ) ;
#3386=CARTESIAN_POINT ( 'NONE',  ( -8.201440678128605555, 5.289679325232168772, 10.00000000000000000 ) ) ;
#3388=CARTESIAN_POINT ( 'NONE',  ( 4.163410377374355598, -12.26152398776834040, 3.747395293195558847E-16 ) ) ;
#3405=CARTESIAN_POINT ( 'NONE',  ( 3.534825977509327366, -7.171832907601992879, 10.00000000000000000 ) ) ;
#3406=CARTESIAN_POINT ( 'NONE',  ( 6.986659217179107095, 9.748146710219840472, 6.857782953271941950E-17 ) ) ;
#3407=PRESENTATION_STYLE_ASSIGNMENT (( #11779 ) ) ;
#3415=CARTESIAN_POINT ( 'NONE',  ( -13.29946171776686903, 6.562258890817373569, 10.00000000000000000 ) ) ;
#3420=CARTESIAN_POINT ( 'NONE',  ( 5.892341078160108658, -4.186101517074008349, 3.747395293195558847E-16 ) ) ;
#3427=CARTESIAN_POINT ( 'NONE',  ( 0.3190826481552657135, -3.778307095988849618, 10.00000000000000000 ) ) ;
#3435=CARTESIAN_POINT ( 'NONE',  ( -6.589974825828272209, 7.038139701356662670, 6.857782953271941950E-17 ) ) ;
#3439=CARTESIAN_POINT ( 'NONE',  ( -3.663109177303994546, -5.348850660921632638, 10.00000000000000000 ) ) ;
#3440=ORIENTED_EDGE ( 'NONE', *, *, #9025, .T. ) ;
#3445=CARTESIAN_POINT ( 'NONE',  ( -1.916691774771272172, -10.52688368019216725, 10.00000000000000000 ) ) ;
#3447=CARTESIAN_POINT ( 'NONE',  ( -2.069312577552832266, -12.54440658741723880, 3.747395293195558847E-16 ) ) ;
#3450=VERTEX_POINT ( 'NONE', #3453 ) ;
#3453=CARTESIAN_POINT ( 'NONE',  ( 16.50000000000000000, 0.000000000000000000, 3.747395293195558847E-16 ) ) ;
#3457=CARTESIAN_POINT ( 'NONE',  ( 0.9209971296404340091, -6.773236541304579639, 3.747395293195558847E-16 ) ) ;
#3465=CARTESIAN_POINT ( 'NONE',  ( -3.764233030011072678, -6.516208816467838894, 10.00000000000000000 ) ) ;
#3466=CARTESIAN_POINT ( 'NONE',  ( 3.343943643650757913, -10.41127694127634129, 6.857782953271941950E-17 ) ) ;
#3472=CARTESIAN_POINT ( 'NONE',  ( -11.98301361336074500, 0.7816210414391656647, 10.00000000000000000 ) ) ;
#3476=CARTESIAN_POINT ( 'NONE',  ( -3.038216613429991053, 4.635879136410029133, 3.747395293195558847E-16 ) ) ;
#3485=CARTESIAN_POINT ( 'NONE',  ( 4.516389116325776776, 1.247036727255508737, 10.00000000000000000 ) ) ;
#3492=CARTESIAN_POINT ( 'NONE',  ( -5.152979166089614260, -5.321787192520350374, 6.857782953271941950E-17 ) ) ;
#3498=CARTESIAN_POINT ( 'NONE',  ( -0.4771094043438766641, 5.286185534804332065, 10.00000000000000000 ) ) ;
#3506=CARTESIAN_POINT ( 'NONE',  ( -0.1504880127287666625, 9.287785325659767111, 10.00000000000000000 ) ) ;
#3514=CARTESIAN_POINT ( 'NONE',  ( 4.516389116325773223, 1.247036727255508515, 3.747395293195558847E-16 ) ) ;
#3520=CARTESIAN_POINT ( 'NONE',  ( 5.267519402444160725, 2.381954139586888175, 10.00000000000000000 ) ) ;
#3521=CARTESIAN_POINT ( 'NONE',  ( -9.352287007201468327, 3.176141031410556703, 6.857782953271941950E-17 ) ) ;
#3528=CARTESIAN_POINT ( 'NONE',  ( 13.54728169684850414, 0.8932250400876640128, 10.00000000000000000 ) ) ;
#3533=CARTESIAN_POINT ( 'NONE',  ( -1.515734900794040385, 8.225284064336934264, 3.747395293195558847E-16 ) ) ;
#3550=CARTESIAN_POINT ( 'NONE',  ( 2.004495162477540671, 5.838205294495789843, 6.857782953271941950E-17 ) ) ;
#3558=CARTESIAN_POINT ( 'NONE',  ( -0.7379871813790722657, -6.677365878963855472, 10.00000000000000000 ) ) ;
#3567=CARTESIAN_POINT ( 'NONE',  ( 17.49999999999999645, 0.000000000000000000, 6.857782953271941950E-17 ) ) ;
#3575=CARTESIAN_POINT ( 'NONE',  ( 0.3190826481552654914, -3.778307095988950870, 3.747395293195558847E-16 ) ) ;
#3580=CARTESIAN_POINT ( 'NONE',  ( -5.101271054653082615, -15.85638610327791476, 10.00000000000000000 ) ) ;
#3582=CARTESIAN_POINT ( 'NONE',  ( -2.682496113117365244, -7.114254743909630641, 6.857782953271941950E-17 ) ) ;
#3590=CARTESIAN_POINT ( 'NONE',  ( -12.61273389267918610, -8.731886703670456384, 10.00000000000000000 ) ) ;
#3595=CARTESIAN_POINT ( 'NONE',  ( 3.678979105947487671, -2.215585777442455662, 3.747395293195558847E-16 ) ) ;
#3604=CARTESIAN_POINT ( 'NONE',  ( 4.340769014460005515, -0.9713985772308084687, 10.00000000000000000 ) ) ;
#3618=CARTESIAN_POINT ( 'NONE',  ( 7.357672848543034050, 2.125097602832379806, 10.00000000000000000 ) ) ;
#3624=CARTESIAN_POINT ( 'NONE',  ( -15.56595607421883365, -4.438723023272252100, 6.857782953271941950E-17 ) ) ;
#3632=CARTESIAN_POINT ( 'NONE',  ( -5.069009347565034851, 2.772702716244574095, 3.747395293195558847E-16 ) ) ;
#3639=CARTESIAN_POINT ( 'NONE',  ( 15.92723891616543774, -6.911623607273383207, 10.00000000000000000 ) ) ;
#3641=CARTESIAN_POINT ( 'NONE',  ( 2.004495162477540671, 5.838205294495789843, 6.857782953271941950E-17 ) ) ;
#3648=CARTESIAN_POINT ( 'NONE',  ( 8.429646098664189680, -5.822225404888640377, 10.00000000000000000 ) ) ;
#3651=CARTESIAN_POINT ( 'NONE',  ( -8.694522232909450921, -2.966707450564700199, 3.747395293195558847E-16 ) ) ;
#3652=CARTESIAN_POINT ( 'NONE',  ( 4.525508228541170297, -0.2388087992699348128, 3.747395293195558847E-16 ) ) ;
#3663=CARTESIAN_POINT ( 'NONE',  ( 12.25096627321951814, 6.291700371256212065, 3.747395293195558847E-16 ) ) ;
#3664=CARTESIAN_POINT ( 'NONE',  ( -0.2556890074706221205, -7.756263830888991961, 6.857782953271941950E-17 ) ) ;
#3673=CARTESIAN_POINT ( 'NONE',  ( -5.541928854458318732, -2.884958602215172974, 10.00000000000000000 ) ) ;
#3680=CARTESIAN_POINT ( 'NONE',  ( -6.451445390047177320, -3.308750875808899483, 10.00000000000000000 ) ) ;
#3690=CARTESIAN_POINT ( 'NONE',  ( 7.195390336726608105, 2.736402267197653337, 3.747395293195558847E-16 ) ) ;
#3697=CARTESIAN_POINT ( 'NONE',  ( 10.64229886435067840, -13.41933351754447834, 10.00000000000000000 ) ) ;
#3706=CARTESIAN_POINT ( 'NONE',  ( -8.984113827416489784, -1.502549133976348816, 10.00000000000000000 ) ) ;
#3713=CARTESIAN_POINT ( 'NONE',  ( -6.597323627731391582, 9.514359934151556786, 3.747395293195558847E-16 ) ) ;
#3726=CARTESIAN_POINT ( 'NONE',  ( -14.24631147015001886, -5.364320868109360596, 3.747395293195558847E-16 ) ) ;
#3727=CARTESIAN_POINT ( 'NONE',  ( 6.689389171169558779, -4.795626085247174153, 6.857782953271941950E-17 ) ) ;
#3744=CARTESIAN_POINT ( 'NONE',  ( -13.43906451854462603, -9.301052350413224090, 6.857782953271941950E-17 ) ) ;
#3755=CARTESIAN_POINT ( 'NONE',  ( 15.00667705184754119, -6.512453894250635145, 10.00000000000000000 ) ) ;
#3763=CARTESIAN_POINT ( 'NONE',  ( -1.103316172498668202, -16.73802372459124754, 10.00000000000000000 ) ) ;
#3764=CARTESIAN_POINT ( 'NONE',  ( 1.018538006779708738, -7.771884277300779686, 6.857782953271941950E-17 ) ) ;
#3768=AXIS2_PLACEMENT_3D ( 'NONE', #11272, #1845, #3923 ) ;
#3774=CARTESIAN_POINT ( 'NONE',  ( 1.831757423467613277, 7.960349185506228942, 10.00000000000000000 ) ) ;
#3779=CARTESIAN_POINT ( 'NONE',  ( -8.962830026514755133, 0.7152994853347065529, 3.747395293195558847E-16 ) ) ;
#3796=CARTESIAN_POINT ( 'NONE',  ( 12.15471013770256903, -5.500887282572993975, 3.747395293195558847E-16 ) ) ;
#3809=CARTESIAN_POINT ( 'NONE',  ( 5.531377455021724288, -0.3672033614207039776, 10.00000000000000000 ) ) ;
#3811=FACE_OUTER_BOUND ( 'NONE', #6615, .T. ) ;
#3817=CARTESIAN_POINT ( 'NONE',  ( 11.72652038055310086, 7.297668919378235586, 10.00000000000000000 ) ) ;
#3818=CARTESIAN_POINT ( 'NONE',  ( 0.0002901587068756704066, -4.749354241797638210, 6.857782953271941950E-17 ) ) ;
#3822=CARTESIAN_POINT ( 'NONE',  ( -9.080917052262543976, 12.68274194616037853, 10.00000000000000000 ) ) ;
#3834=CARTESIAN_POINT ( 'NONE',  ( -9.037587479195734019, -0.7561632655184234997, 10.00000000000000000 ) ) ;
#3837=CARTESIAN_POINT ( 'NONE',  ( -5.920784292472551336, 6.290491683487165808, 3.747395293195558847E-16 ) ) ;
#3838=CARTESIAN_POINT ( 'NONE',  ( 0.3190826481552654914, -3.778307095988950870, 3.747395293195558847E-16 ) ) ;
#3851=CARTESIAN_POINT ( 'NONE',  ( 6.600721363681633314, -14.58171973507987396, 3.747395293195558847E-16 ) ) ;
#3863=CARTESIAN_POINT ( 'NONE',  ( -8.799721882313772170, 9.100398320382241835, 6.857782953271941950E-17 ) ) ;
#3870=VERTEX_POINT ( 'NONE', #7086 ) ;
#3871=CARTESIAN_POINT ( 'NONE',  ( -14.60057116351880069, -4.165219547604622541, 10.00000000000000000 ) ) ;
#3873=( LENGTH_UNIT ( ) NAMED_UNIT ( * ) SI_UNIT ( .MILLI., .METRE. ) );
#3878=CARTESIAN_POINT ( 'NONE',  ( 4.451863640886955409, 11.26298505921346305, 10.00000000000000000 ) ) ;
#3887=CARTESIAN_POINT ( 'NONE',  ( 6.685168693379562654, -7.607270790100137958, 10.00000000000000000 ) ) ;
#3891=CARTESIAN_POINT ( 'NONE',  ( 0.5199114366211738947, 8.229807867079655281, 3.747395293195558847E-16 ) ) ;
#3893=CARTESIAN_POINT ( 'NONE',  ( 14.22875512193218661, -2.589574901423981057, 6.857782953271941950E-17 ) ) ;
#3906=CARTESIAN_POINT ( 'NONE',  ( -14.61026919807147095, 3.159152207411756397, 3.747395293195558847E-16 ) ) ;
#3916=CARTESIAN_POINT ( 'NONE',  ( 1.445324715877977173, -3.701599742324200637, 10.00000000000000000 ) ) ;
#3923=DIRECTION ( 'NONE',  ( 1.000000000000000000, 0.000000000000000000, 0.000000000000000000 ) ) ;
#3924=CARTESIAN_POINT ( 'NONE',  ( 13.14573027368987646, 6.745762002080606834, 6.857782953271941950E-17 ) ) ;
#3925=PLANE ( 'NONE',  #2365 ) ;
#3935=CARTESIAN_POINT ( 'NONE',  ( 7.081399987883182590, -10.98142027556026967, 10.00000000000000000 ) ) ;
#3944=CARTESIAN_POINT ( 'NONE',  ( -12.98359546555290045, 0.8565524458112724338, 10.00000000000000000 ) ) ;
#3953=CARTESIAN_POINT ( 'NONE',  ( -1.790740696106539520, -6.394195405909708363, 10.00000000000000000 ) ) ;
#3955=CARTESIAN_POINT ( 'NONE',  ( 8.143984375790578767, 3.063465613658708619, 10.00000000000000000 ) ) ;
#3957=CARTESIAN_POINT ( 'NONE',  ( -12.91830213043053988, -2.344901317288421883, 6.857782953271941950E-17 ) ) ;
#3969=CARTESIAN_POINT ( 'NONE',  ( -11.98301361336074145, 0.7816210414391653316, 3.747395293195558847E-16 ) ) ;
#3979=CARTESIAN_POINT ( 'NONE',  ( -11.98007164540817371, 10.17225797950328214, 10.00000000000000000 ) ) ;
#3988=CARTESIAN_POINT ( 'NONE',  ( -8.211874628637438889, -10.69266484962706087, 6.857782953271941950E-17 ) ) ;
#3996=CARTESIAN_POINT ( 'NONE',  ( -14.24631147015002242, -5.364320868108786833, 10.00000000000000000 ) ) ;
#4001=CARTESIAN_POINT ( 'NONE',  ( 11.51680056346192593, -0.3781118375584788249, 10.00000000000000000 ) ) ;
#4003=CARTESIAN_POINT ( 'NONE',  ( -8.207979594962566239, -13.19054478262514252, 3.747395293195558847E-16 ) ) ;
#4012=CARTESIAN_POINT ( 'NONE',  ( -3.663109177303994546, -5.348850660921632638, 10.00000000000000000 ) ) ;
#4014=CARTESIAN_POINT ( 'NONE',  ( 10.63538685525201188, -4.008487272325480966, 10.00000000000000000 ) ) ;
#4015=CARTESIAN_POINT ( 'NONE',  ( 12.58137556868280882, 7.823023050434559700, 6.857782953271941950E-17 ) ) ;
#4024=CARTESIAN_POINT ( 'NONE',  ( 4.889075487039526990, 9.929493272050624597, 3.747395293195558847E-16 ) ) ;
#4030=CARTESIAN_POINT ( 'NONE',  ( -3.251399079312189855, 15.05603916236422890, 10.00000000000000000 ) ) ;
#4043=CARTESIAN_POINT ( 'NONE',  ( 0.5005346673319864825, 15.27733729710887545, 6.857782953271941950E-17 ) ) ;
#4048=ORIENTED_EDGE ( 'NONE', *, *, #12012, .F. ) ;
#4049=CARTESIAN_POINT ( 'NONE',  ( 5.319643049700913728, -8.526005966359200272, 10.00000000000000000 ) ) ;
#4055=CARTESIAN_POINT ( 'NONE',  ( 4.479449988082535583, -13.21383449271838550, 10.00000000000000000 ) ) ;
#4058=CARTESIAN_POINT ( 'NONE',  ( -14.85975435031504510, 1.953672781916663936, 3.747395293195558847E-16 ) ) ;
#4068=CARTESIAN_POINT ( 'NONE',  ( -3.231136241382285501, -5.666136714101813965, 10.00000000000000000 ) ) ;
#4071=CARTESIAN_POINT ( 'NONE',  ( 10.90031251054716499, 4.301772984117411269, 10.00000000000000000 ) ) ;
#4072=CARTESIAN_POINT ( 'NONE',  ( -2.240087900411201982, -13.53314956822677928, 6.857782953271941950E-17 ) ) ;
#4087=CARTESIAN_POINT ( 'NONE',  ( 2.355103038863950893, 10.93470652055903791, 3.747395293195558847E-16 ) ) ;
#4092=CARTESIAN_POINT ( 'NONE',  ( 7.525577113297165610, 13.03378399180780889, 10.00000000000000000 ) ) ;
#4101=CARTESIAN_POINT ( 'NONE',  ( -11.98007164540816838, 10.17225797950327681, 6.857782953271941950E-17 ) ) ;
#4109=CARTESIAN_POINT ( 'NONE',  ( 3.053028024665676021, -9.450988318042126579, 10.00000000000000000 ) ) ;
#4116=CARTESIAN_POINT ( 'NONE',  ( -7.159234172427928478, 10.34564589702411475, 10.00000000000000000 ) ) ;
#4120=CARTESIAN_POINT ( 'NONE',  ( -9.470608727120474413, 11.15741021143934297, 3.747395293195558847E-16 ) ) ;
#4124=STYLED_ITEM ( 'NONE', ( #10717 ), #7312 ) ;
#4136=CARTESIAN_POINT ( 'NONE',  ( -4.625218816435448410, 8.325684435358759572, 10.00000000000000000 ) ) ;
#4137=CARTESIAN_POINT ( 'NONE',  ( -6.864300873105353418, 13.92024697337931549, 6.857782953271941950E-17 ) ) ;
#4153=CARTESIAN_POINT ( 'NONE',  ( -3.937910939466568117, -8.732312745279397603, 3.747395293195558847E-16 ) ) ;
#4158=CARTESIAN_POINT ( 'NONE',  ( 4.479449988082535583, -13.21383449271838550, 10.00000000000000000 ) ) ;
#4165=VERTEX_POINT ( 'NONE', #5872 ) ;
#4169=CARTESIAN_POINT ( 'NONE',  ( -5.965338750500049692, 7.524205049158500636, 6.857782953271941950E-17 ) ) ;
#4175=CARTESIAN_POINT ( 'NONE',  ( -9.037587479195734019, -0.7561632655184234997, 10.00000000000000000 ) ) ;
#4181=CARTESIAN_POINT ( 'NONE',  ( 5.835571643920557605, -9.386589068694828342, 10.00000000000000000 ) ) ;
#4184=CARTESIAN_POINT ( 'NONE',  ( -1.036640877615904843, -15.73686152240404468, 3.747395293195558847E-16 ) ) ;
#4194=CARTESIAN_POINT ( 'NONE',  ( 6.396238541183701720, 6.183590428399974748, 10.00000000000000000 ) ) ;
#4195=CARTESIAN_POINT ( 'NONE',  ( 5.027256439335598515, -9.798587832408038878, 6.857782953271941950E-17 ) ) ;
#4206=CARTESIAN_POINT ( 'NONE',  ( -10.73274959028096198, -5.974010873319483217, 3.747395293195558847E-16 ) ) ;
#4211=EDGE_CURVE ( 'NONE', #5043, #1562, #4537, .T. ) ;
#4212=CARTESIAN_POINT ( 'NONE',  ( -7.159234172427928478, 10.34564589702411475, 10.00000000000000000 ) ) ;
#4222=CARTESIAN_POINT ( 'NONE',  ( 8.025946968469181542, -7.769110617520081696, 6.857782953271941950E-17 ) ) ;
#4229=CARTESIAN_POINT ( 'NONE',  ( 8.282588618526579793, 7.043362411858248073, 10.00000000000000000 ) ) ;
#4236=CARTESIAN_POINT ( 'NONE',  ( 8.393308867179015920, -1.106660293010312657, 10.00000000000000000 ) ) ;
#4239=CARTESIAN_POINT ( 'NONE',  ( 12.15471013770256903, -5.500887282572993975, 3.747395293195558847E-16 ) ) ;
#4248=CARTESIAN_POINT ( 'NONE',  ( -3.542987847618590536, 5.503081486278161627, 10.00000000000000000 ) ) ;
#4249=CARTESIAN_POINT ( 'NONE',  ( -1.672018190274121574, 9.216430685901386255, 6.857782953271941950E-17 ) ) ;
#4257=CARTESIAN_POINT ( 'NONE',  ( -13.83044629298881389, 5.462350471645223138, 10.00000000000000000 ) ) ;
#4261=CARTESIAN_POINT ( 'NONE',  ( 5.498207398720008854, -4.630339417915828371, 3.747395293195558847E-16 ) ) ;
#4268=CARTESIAN_POINT ( 'NONE',  ( 8.588976300537440878, -11.19439025337201343, 10.00000000000000000 ) ) ;
#4271=CARTESIAN_POINT ( 'NONE',  ( -3.038216613430223756, 4.635879136410493651, 10.00000000000000000 ) ) ;
#4279=CARTESIAN_POINT ( 'NONE',  ( -1.410059164928062048, 12.26527237696109474, 6.857782953271941950E-17 ) ) ;
#4284=CARTESIAN_POINT ( 'NONE',  ( -10.73274959028002229, -5.974010873319484105, 10.00000000000000000 ) ) ;
#4292=CARTESIAN_POINT ( 'NONE',  ( -9.386162357322616501, -4.067606288967439809, 10.00000000000000000 ) ) ;
#4294=CARTESIAN_POINT ( 'NONE',  ( 10.44364468045615801, 9.157203537817473205, 3.747395293195558847E-16 ) ) ;
#4309=CARTESIAN_POINT ( 'NONE',  ( 10.90031251054715966, 4.301772984117409493, 6.857782953271941950E-17 ) ) ;
#4319=CARTESIAN_POINT ( 'NONE',  ( 4.977139221860650942, 13.21892491369670530, 10.00000000000000000 ) ) ;
#4324=CARTESIAN_POINT ( 'NONE',  ( 3.656769781543557141, 7.172433557890304456, 3.747395293195558847E-16 ) ) ;
#4331=CARTESIAN_POINT ( 'NONE',  ( 3.678979105947490780, -2.215585777442456550, 10.00000000000000000 ) ) ;
#4332=ADVANCED_FACE ( 'NONE', ( #11167 ), #10310, .F. ) ;
#4342=CARTESIAN_POINT ( 'NONE',  ( -2.433178163897522506, 9.086443520544598584, 6.857782953271941950E-17 ) ) ;
#4349=CARTESIAN_POINT ( 'NONE',  ( 4.212679447664378074, 6.814025269448781508, 10.00000000000000000 ) ) ;
#4356=CARTESIAN_POINT ( 'NONE',  ( 9.774996403550735735, -5.644905071530105900, 10.00000000000000000 ) ) ;
#4358=CARTESIAN_POINT ( 'NONE',  ( -4.054747718262373901, -11.96785467447665674, 3.747395293195558847E-16 ) ) ;
#4374=CARTESIAN_POINT ( 'NONE',  ( -6.451445390047177320, -3.308750875808899483, 10.00000000000000000 ) ) ;
#4376=CARTESIAN_POINT ( 'NONE',  ( -1.916691774771271284, -10.52688368019216014, 6.857782953271941950E-17 ) ) ;
#4377=DIRECTION ( 'NONE',  ( -6.938893903907228378E-16, -0.000000000000000000, -1.000000000000000000 ) ) ;
#4384=CARTESIAN_POINT ( 'NONE',  ( 9.683839015878914935, 10.01260560230626595, 10.00000000000000000 ) ) ;
#4388=CARTESIAN_POINT ( 'NONE',  ( -4.428608208598374674, -4.627450663480007442, 3.747395293195558847E-16 ) ) ;
#4391=ORIENTED_EDGE ( 'NONE', *, *, #9025, .F. ) ;
#4401=CARTESIAN_POINT ( 'NONE',  ( 6.396238541184324333, 6.183590428399971195, 6.857782953271941950E-17 ) ) ;
#4408=CARTESIAN_POINT ( 'NONE',  ( -1.784247137544766604, 5.123456263349899231, 10.00000000000000000 ) ) ;
#4417=CARTESIAN_POINT ( 'NONE',  ( -7.130211940009574256, -7.605417807865423541, 10.00000000000000000 ) ) ;
#4425=CARTESIAN_POINT ( 'NONE',  ( -6.012500708481076650, 0.06204199954272016787, 3.747395293195558847E-16 ) ) ;
#4432=CARTESIAN_POINT ( 'NONE',  ( -2.682496113117368797, -7.114254743909099510, 10.00000000000000000 ) ) ;
#4434=CARTESIAN_POINT ( 'NONE',  ( -1.410059164928062048, 12.26527237696109474, 6.857782953271941950E-17 ) ) ;
#4439=EDGE_LOOP ( 'NONE', ( #4391, #6018, #5857, #2953 ) ) ;
#4440=CARTESIAN_POINT ( 'NONE',  ( -9.470608727121586412, 11.15741021143934653, 10.00000000000000000 ) ) ;
#4444=CARTESIAN_POINT ( 'NONE',  ( 6.841929108544086091, -2.672872603904024480, 3.747395293195558847E-16 ) ) ;
#4453=CARTESIAN_POINT ( 'NONE',  ( -4.158472309566741743, 3.840014155104743754, 10.00000000000000000 ) ) ;
#4460=CARTESIAN_POINT ( 'NONE',  ( -4.006926059188537614, 5.225193401749451461, 6.857782953271941950E-17 ) ) ;
#4466=CARTESIAN_POINT ( 'NONE',  ( 5.498207398719435091, -4.630339417915830147, 10.00000000000000000 ) ) ;
#4474=CARTESIAN_POINT ( 'NONE',  ( -4.006926059189011902, 5.225193401749456790, 10.00000000000000000 ) ) ;
#4483=CARTESIAN_POINT ( 'NONE',  ( 4.340769014460001962, -0.9713985772308075806, 3.747395293195558847E-16 ) ) ;
#4493=CARTESIAN_POINT ( 'NONE',  ( -2.061894914253512123, 6.087690860853031793, 6.857782953271941950E-17 ) ) ;
#4497=CARTESIAN_POINT ( 'NONE',  ( 0.0002901587068752367257, -4.749354241797645315, 10.00000000000000000 ) ) ;
#4503=CARTESIAN_POINT ( 'NONE',  ( -10.19073739998278683, -11.62312336453203798, 10.00000000000000000 ) ) ;
#4507=CARTESIAN_POINT ( 'NONE',  ( 4.623190192904133689, -5.402202315098909580, 3.747395293195558847E-16 ) ) ;
#4533=EDGE_CURVE ( 'NONE', #5043, #1474, #5173, .T. ) ;
#4537=B_SPLINE_CURVE_WITH_KNOTS ( 'NONE', 3,
 ( #7637, #349, #10335, #8569, #10400, #9424, #3117, #2131, #9662, #11383, #9602, #233, #3002, #2076, #1045, #4892, #6777, #1954, #7575, #4958, #5813, #5757, #8630, #4774, #293, #9541, #9482, #1221, #8513, #1279, #1156, #167, #3979, #111, #6836, #8695, #7704, #4030, #7758, #10580, #2196, #5936, #5012, #4092, #7822, #11559, #1398, #7941, #2256, #5992, #473, #3233, #5132, #10643, #2435, #9775, #11616, #8926, #7995, #4268, #6900, #7010, #4158, #8982, #5248, #8871, #3181, #11733, #595, #7886, #5191, #11670, #6953, #533, #9717, #1456, #3357, #6113, #1331, #7071, #9901, #5067, #10825, #6174, #413, #4212, #3288, #10697, #8807, #10757, #6047, #2309, #2373, #9846, #1515, #2234, #10679, #9583, #10554, #11477, #4071, #6879, #2291, #272, #10621, #4993, #4014, #3097, #10438, #9641, #7800, #11356, #8610, #9700, #7740, #6815, #2173, #3160, #8785, #5852, #6933, #11537, #2056, #6027, #5914, #11421, #1261, #1135, #7866, #5970, #2980, #1312, #8731, #333, #5048, #391, #9755, #4136, #5794, #11599, #4871, #5106, #3216, #1375, #8850, #9519, #3042, #454, #4194, #6701, #206, #3955, #7682, #6760, #10496, #2112, #1197, #4935, #8672, #11776, #11653, #8907, #10060, #3405, #513, #640, #9089, #9140, #2603, #6272, #4432, #3465, #6091, #2350, #11891, #10985, #4374, #1555, #3269, #10804, #7052, #6991, #2414, #698, #5170, #10736, #9882, #5292, #4248, #10917, #7232, #1679, #7173, #5360, #7920, #7975, #8164, #3520, #1438, #8108, #1624, #11710, #5414, #756, #9822, #11833, #2534, #9998 ),
 .UNSPECIFIED., .F., .F.,
 ( 4, 2, 2, 2, 2, 2, 2, 2, 2, 2, 2, 2, 2, 2, 2, 2, 2, 2, 2, 2, 2, 2, 2, 2, 2, 2, 2, 2, 2, 2, 2, 2, 2, 2, 2, 2, 2, 2, 2, 2, 2, 2, 2, 2, 2, 2, 2, 2, 2, 2, 2, 2, 2, 2, 2, 2, 2, 2, 2, 2, 2, 2, 2, 2, 2, 2, 2, 2, 2, 2, 2, 2, 2, 2, 2, 2, 2, 2, 2, 2, 2, 2, 2, 2, 2, 2, 2, 2, 2, 2, 2, 2, 2, 2, 2, 2, 2, 2, 2, 2, 2, 2, 2, 4 ),
 ( 0.000000000000000000, 0.007812500000000000000, 0.01562500000000000000, 0.02343750000000000000, 0.03125000000000000000, 0.03906250000000000000, 0.04687500000000000000, 0.05468750000000000000, 0.06250000000000000000, 0.07031250000000000000, 0.07812500000000000000, 0.08593750000000000000, 0.09375000000000000000, 0.1015624999999999861, 0.1093750000000000000, 0.1171875000000000000, 0.1250000000000000000, 0.1328125000000000000, 0.1406250000000000000, 0.1484375000000000000, 0.1562500000000000000, 0.1640624999999999722, 0.1718750000000000000, 0.1796875000000000000, 0.1875000000000000000, 0.1953125000000000000, 0.2031249999999999722, 0.2109375000000000000, 0.2187500000000000000, 0.2265625000000000000, 0.2343750000000000000, 0.2421875000000000000, 0.2500000000000000000, 0.2578125000000000000, 0.2656250000000000000, 0.2734375000000000000, 0.2812500000000000000, 0.2890625000000000000, 0.2968750000000000000, 0.3046875000000000000, 0.3125000000000000000, 0.3203125000000000000, 0.3281249999999999445, 0.3359375000000000000, 0.3437500000000000000, 0.3515625000000000000, 0.3593750000000000000, 0.3671874999999999445, 0.3750000000000000000, 0.3828125000000000000, 0.3906250000000000000, 0.3984375000000000000, 0.4062499999999999445, 0.4140625000000000000, 0.4218750000000000000, 0.4296875000000000000, 0.4375000000000000000, 0.4453125000000000000, 0.4531250000000000000, 0.4609375000000000000, 0.4687500000000000000, 0.4765625000000000000, 0.4843750000000000000, 0.4921875000000000000, 0.5000000000000000000, 0.5078125000000000000, 0.5156250000000000000, 0.5234375000000000000, 0.5312500000000000000, 0.5390625000000000000, 0.5468750000000000000, 0.5546875000000000000, 0.5625000000000000000, 0.5703125000000000000, 0.5781250000000000000, 0.5859375000000000000, 0.5937500000000000000, 0.6015625000000000000, 0.6093750000000000000, 0.6171874999999998890, 0.6250000000000000000, 0.6328125000000000000, 0.6406250000000000000, 0.6484375000000000000, 0.6562499999999998890, 0.6640625000000000000, 0.6718750000000000000, 0.6796875000000000000, 0.6875000000000000000, 0.6953124999999998890, 0.7031250000000000000, 0.7109375000000000000, 0.7187500000000000000, 0.7265625000000000000, 0.7343749999999998890, 0.7421875000000000000, 0.7500000000000000000, 0.7656250000000000000, 0.7812500000000000000, 0.7968750000000000000, 0.8124999999999998890, 0.8281250000000000000, 0.8437500000000000000, 0.8499999999999999778 ),
 .UNSPECIFIED. ) ;
#4538=CARTESIAN_POINT ( 'NONE',  ( 0.5199114366211746718, 8.229807867079658834, 10.00000000000000000 ) ) ;
#4546=CARTESIAN_POINT ( 'NONE',  ( -10.85385039129052842, -12.37615246896657339, 6.857782953271941950E-17 ) ) ;
#4554=CARTESIAN_POINT ( 'NONE',  ( 7.261170810407326037, -1.543028577657243439, 3.747395293195558847E-16 ) ) ;
#4559=CARTESIAN_POINT ( 'NONE',  ( 0.6279411196271849072, -4.781877258324066737, 6.857782953271941950E-17 ) ) ;
#4569=CARTESIAN_POINT ( 'NONE',  ( 9.701579622838506722, -3.641351606116563389, 10.00000000000000000 ) ) ;
#4574=CARTESIAN_POINT ( 'NONE',  ( -8.457858257354885723, -3.686763380685289970, 3.747395293195558847E-16 ) ) ;
#4584=CARTESIAN_POINT ( 'NONE',  ( 0.07364157424580693168, -3.751631698233777179, 5.000000000000000000 ) ) ;
#4589=CARTESIAN_POINT ( 'NONE',  ( -9.470608727120474413, 11.15741021143934297, 3.747395293195558847E-16 ) ) ;
#4590=CARTESIAN_POINT ( 'NONE',  ( 5.247589697392725405, -6.187652788349031319, 6.857782953271941950E-17 ) ) ;
#4599=CARTESIAN_POINT ( 'NONE',  ( 6.841929108544089644, -2.672872603903728717, 10.00000000000000000 ) ) ;
#4606=CARTESIAN_POINT ( 'NONE',  ( -2.570438583093578533, 5.934334910739571534, 10.00000000000000000 ) ) ;
#4614=CARTESIAN_POINT ( 'NONE',  ( -5.846204292276366843, 1.022993486932169516, 3.747395293195558847E-16 ) ) ;
#4621=MANIFOLD_SOLID_BREP ( 'Sweep1', #6859 ) ;
#4622=CARTESIAN_POINT ( 'NONE',  ( 1.022653496104248605, 6.171874473422422902, 6.857782953271941950E-17 ) ) ;
#4629=CARTESIAN_POINT ( 'NONE',  ( -4.046710180314750716, 10.72208681399755648, 10.00000000000000000 ) ) ;
#4632=CARTESIAN_POINT ( 'NONE',  ( 4.583115687978880359, -8.898851689028539624, 3.747395293195558847E-16 ) ) ;
#4633=CARTESIAN_POINT ( 'NONE',  ( 0.07364157424580704270, -3.751631698233870438, 3.747395293195558847E-16 ) ) ;
#4646=CARTESIAN_POINT ( 'NONE',  ( 0.2599977045009999599, -15.80854529698373589, 3.747395293195558847E-16 ) ) ;
#4647=CARTESIAN_POINT ( 'NONE',  ( -3.542987847618818353, 5.503081486278154522, 6.857782953271941950E-17 ) ) ;
#4659=PLANE ( 'NONE',  #9705 ) ;
#4663=CARTESIAN_POINT ( 'NONE',  ( -5.248573321596930796, 4.168074790661433049, 10.00000000000000000 ) ) ;
#4672=CARTESIAN_POINT ( 'NONE',  ( -1.035167565893234443, -12.71157708251009488, 10.00000000000000000 ) ) ;
#4677=CARTESIAN_POINT ( 'NONE',  ( 7.014224211608842907, -15.49593329755746929, 10.00000000000000000 ) ) ;
#4679=CARTESIAN_POINT ( 'NONE',  ( -6.661525743073264394, 1.789546221321740793, 6.857782953271941950E-17 ) ) ;
#4688=CARTESIAN_POINT ( 'NONE',  ( -0.1481022647113163504, -9.773457036294484368, 10.00000000000000000 ) ) ;
#4693=CARTESIAN_POINT ( 'NONE',  ( -7.812220363925484357, -5.053636123081432174, 3.747395293195558847E-16 ) ) ;
#4710=CARTESIAN_POINT ( 'NONE',  ( 7.983652613117083519, -10.39416588708253819, 3.747395293195558847E-16 ) ) ;
#4730=CARTESIAN_POINT ( 'NONE',  ( 16.47843063274904196, -5.593696103119284224, 6.857782953271941950E-17 ) ) ;
#4732=DIRECTION ( 'NONE',  ( -0.9973083954695386444, 0.07332096784668425127, 7.625284521749261502E-18 ) ) ;
#4738=CARTESIAN_POINT ( 'NONE',  ( 4.123629756450001516, -15.38522696314584870, 10.00000000000000000 ) ) ;
#4742=CARTESIAN_POINT ( 'NONE',  ( -5.683926142426734884, 14.39978054689284193, 10.00000000000000000 ) ) ;
#4743=CARTESIAN_POINT ( 'NONE',  ( 4.346347989803176937, 4.041826679702269942, 6.857782953271941950E-17 ) ) ;
#4753=CARTESIAN_POINT ( 'NONE',  ( -8.457858257355617582, -3.686763380685291747, 10.00000000000000000 ) ) ;
#4756=CARTESIAN_POINT ( 'NONE',  ( -2.487495860704069361, -9.331140650584718088, 3.747395293195558847E-16 ) ) ;
#4770=CARTESIAN_POINT ( 'NONE',  ( 13.53515989517831564, -0.2218654272304620700, 3.747395293195558847E-16 ) ) ;
#4774=CARTESIAN_POINT ( 'NONE',  ( -15.18624859168667918, -5.715447929355455869, 10.00000000000000000 ) ) ;
#4782=CARTESIAN_POINT ( 'NONE',  ( -11.39998097177137026, 5.856612080558655897, 6.857782953271941950E-17 ) ) ;
#4793=CARTESIAN_POINT ( 'NONE',  ( -14.61026919807147451, 3.159152207411757285, 10.00000000000000000 ) ) ;
#4798=CARTESIAN_POINT ( 'NONE',  ( -0.3972327064967878796, 12.29993208790120640, 10.00000000000000000 ) ) ;
#4801=CARTESIAN_POINT ( 'NONE',  ( -5.101271054653079950, -15.85638610327790765, 6.857782953271941950E-17 ) ) ;
#4808=CARTESIAN_POINT ( 'NONE',  ( 8.913847851856345983, -5.129921849437908854, 10.00000000000000000 ) ) ;
#4812=CARTESIAN_POINT ( 'NONE',  ( -0.1481022647113159063, -9.773457036294480815, 3.747395293195558847E-16 ) ) ;
#4813=CARTESIAN_POINT ( 'NONE',  ( 0.5005346673319864825, 15.27733729710887545, 6.857782953271941950E-17 ) ) ;
#4825=CARTESIAN_POINT ( 'NONE',  ( -1.872083171988683015, 14.23747171912756038, 3.747395293195558847E-16 ) ) ;
#4826=ADVANCED_FACE ( 'NONE', ( #2225 ), #6595, .F. ) ;
#4839=CARTESIAN_POINT ( 'NONE',  ( 14.54887842078032278, 0.9530482589069305677, 6.857782953271941950E-17 ) ) ;
#4847=CARTESIAN_POINT ( 'NONE',  ( 7.983652613117085295, -10.39416588708253997, 10.00000000000000000 ) ) ;
#4850=CARTESIAN_POINT ( 'NONE',  ( 15.92723891616420673, -6.911623607273379655, 6.857782953271941950E-17 ) ) ;
#4854=CARTESIAN_POINT ( 'NONE',  ( -1.410059164928063380, 12.26527237696110184, 10.00000000000000000 ) ) ;
#4856=CARTESIAN_POINT ( 'NONE',  ( -7.115032382426029756, -13.85544350050026452, 3.747395293195558847E-16 ) ) ;
#4867=CARTESIAN_POINT ( 'NONE',  ( 6.841929108544089644, -2.672872603903728717, 10.00000000000000000 ) ) ;
#4871=CARTESIAN_POINT ( 'NONE',  ( -1.672018190274039418, 9.216430685901391584, 10.00000000000000000 ) ) ;
#4873=CARTESIAN_POINT ( 'NONE',  ( 14.54887842078032278, 0.9530482589069305677, 6.857782953271941950E-17 ) ) ;
#4881=CARTESIAN_POINT ( 'NONE',  ( -3.562082835880472587, -15.28349083755603743, 10.00000000000000000 ) ) ;
#4887=CARTESIAN_POINT ( 'NONE',  ( -11.74902089294173457, -3.156991809147609906, 3.747395293195558847E-16 ) ) ;
#4892=CARTESIAN_POINT ( 'NONE',  ( -3.791520748785662587, -16.26028641251513207, 10.00000000000000000 ) ) ;
#4904=CARTESIAN_POINT ( 'NONE',  ( -3.406233159845096559, 11.94786423299364486, 6.857782953271941950E-17 ) ) ;
#4913=CARTESIAN_POINT ( 'NONE',  ( -7.115032382426030644, -13.85544350050026807, 10.00000000000000000 ) ) ;
#4920=CARTESIAN_POINT ( 'NONE',  ( 11.37845468071832222, 2.456417158213071161, 10.00000000000000000 ) ) ;
#4922=CARTESIAN_POINT ( 'NONE',  ( 15.52845182490561271, -5.270724383582042094, 3.747395293195558847E-16 ) ) ;
#4931=CARTESIAN_POINT ( 'NONE',  ( -6.036922680726761747, -0.4347383792561346771, 10.00000000000000000 ) ) ;
#4932=LINE ( 'NONE', #11242, #352 ) ;
#4935=CARTESIAN_POINT ( 'NONE',  ( 7.763517025773944980, -3.069710483245354116, 10.00000000000000000 ) ) ;
#4937=CARTESIAN_POINT ( 'NONE',  ( 13.06601448280974509, -5.920767845834311593, 6.857782953271941950E-17 ) ) ;
#4951=CARTESIAN_POINT ( 'NONE',  ( 6.685168693379560878, -7.607270790100919555, 3.747395293195558847E-16 ) ) ;
#4958=CARTESIAN_POINT ( 'NONE',  ( -10.85385039129053197, -12.37615246896657872, 10.00000000000000000 ) ) ;
#4968=CARTESIAN_POINT ( 'NONE',  ( -5.414455899168758357, -12.47541146648942245, 6.857782953271941950E-17 ) ) ;
#4975=CARTESIAN_POINT ( 'NONE',  ( 6.685168693379562654, -7.607270790100137958, 10.00000000000000000 ) ) ;
#4982=CARTESIAN_POINT ( 'NONE',  ( -10.47176928358605075, -8.303818807687077808, 10.00000000000000000 ) ) ;
#4984=CARTESIAN_POINT ( 'NONE',  ( -13.25288834650809555, -7.646628085888695914, 3.747395293195558847E-16 ) ) ;
#4990=CARTESIAN_POINT ( 'NONE',  ( 5.498207398719435091, -4.630339417915830147, 10.00000000000000000 ) ) ;
#4993=CARTESIAN_POINT ( 'NONE',  ( 10.96671743108979058, -3.132869264233008266, 10.00000000000000000 ) ) ;
#4994=CARTESIAN_POINT ( 'NONE',  ( 5.564773995946417529, -12.83798980516507626, 6.857782953271941950E-17 ) ) ;
#5004=CARTESIAN_POINT ( 'NONE',  ( -6.777230418910821896, -10.52530689671158193, 3.747395293195558847E-16 ) ) ;
#5012=CARTESIAN_POINT ( 'NONE',  ( 5.334478431285540445, 14.15651896542077104, 10.00000000000000000 ) ) ;
#5023=CARTESIAN_POINT ( 'NONE',  ( 13.99323099382916169, 4.495563823643927037, 6.857782953271941950E-17 ) ) ;
#5024=PRODUCT_DEFINITION_SHAPE ( 'NONE', 'NONE',  #9275 ) ;
#5029=CARTESIAN_POINT ( 'NONE',  ( -1.719633853164447057, -9.543036404944420070, 10.00000000000000000 ) ) ;
#5031=( LENGTH_UNIT ( ) NAMED_UNIT ( * ) SI_UNIT ( .MILLI., .METRE. ) );
#5035=CARTESIAN_POINT ( 'NONE',  ( -8.211874628637442441, -10.69266484962706620, 10.00000000000000000 ) ) ;
#5038=CARTESIAN_POINT ( 'NONE',  ( 7.795318149608630343, -14.02504990431079612, 3.747395293195558847E-16 ) ) ;
#5043=VERTEX_POINT ( 'NONE', #2259 ) ;
#5048=CARTESIAN_POINT ( 'NONE',  ( -7.708066421255711731, 5.920849505456871498, 10.00000000000000000 ) ) ;
#5049=CARTESIAN_POINT ( 'NONE',  ( 5.334478431285537781, 14.15651896542076749, 6.857782953271941950E-17 ) ) ;
#5062=CARTESIAN_POINT ( 'NONE',  ( 10.41236255589546822, -1.188820951657898473, 3.747395293195558847E-16 ) ) ;
#5067=CARTESIAN_POINT ( 'NONE',  ( -11.39998097177319636, 5.856612080558658562, 10.00000000000000000 ) ) ;
#5076=CARTESIAN_POINT ( 'NONE',  ( -10.03906249502028558, -0.8181230654450031281, 6.857782953271941950E-17 ) ) ;
#5084=CARTESIAN_POINT ( 'NONE',  ( -8.457858257355617582, -3.686763380685291747, 10.00000000000000000 ) ) ;
#5091=CARTESIAN_POINT ( 'NONE',  ( -9.960937504979712642, 0.8181230654450121209, 10.00000000000000000 ) ) ;
#5095=CARTESIAN_POINT ( 'NONE',  ( -11.08238827499517321, -10.71925978067678642, 3.747395293195558847E-16 ) ) ;
#5106=CARTESIAN_POINT ( 'NONE',  ( -0.1504880127287666625, 9.287785325659767111, 10.00000000000000000 ) ) ;
#5108=CARTESIAN_POINT ( 'NONE',  ( 11.40744677810890373, -1.317628706759688129, 6.857782953271941950E-17 ) ) ;
#5125=CARTESIAN_POINT ( 'NONE',  ( -8.799590028668786701, 7.703979956834778875, 3.747395293195558847E-16 ) ) ;
#5132=CARTESIAN_POINT ( 'NONE',  ( 14.53830338343600559, -0.2437330612273629071, 10.00000000000000000 ) ) ;
#5141=CARTESIAN_POINT ( 'NONE',  ( 8.143984375791809782, 3.063465613658396425, 6.857782953271941950E-17 ) ) ;
#5149=CARTESIAN_POINT ( 'NONE',  ( -8.799590028668788477, 7.703979956833879150, 10.00000000000000000 ) ) ;
#5154=CARTESIAN_POINT ( 'NONE',  ( 9.246005348854476225, -6.405614325510554430, 10.00000000000000000 ) ) ;
#5157=CARTESIAN_POINT ( 'NONE',  ( -10.73274959028096198, -5.974010873319483217, 3.747395293195558847E-16 ) ) ;
#5170=CARTESIAN_POINT ( 'NONE',  ( -5.924299593718521884, 3.297400215539481039, 10.00000000000000000 ) ) ;
#5172=CARTESIAN_POINT ( 'NONE',  ( -7.708066421255707290, 5.920849505456867945, 6.857782953271941950E-17 ) ) ;
#5173=LINE ( 'NONE', #1498, #7653 ) ;
#5181=CARTESIAN_POINT ( 'NONE',  ( 12.15471013770155295, -5.500887282572486825, 10.00000000000000000 ) ) ;
#5185=CARTESIAN_POINT ( 'NONE',  ( 4.140589500486089314, -5.731468560950439439, 3.747395293195558847E-16 ) ) ;
#5191=CARTESIAN_POINT ( 'NONE',  ( -8.211874628637442441, -10.69266484962706620, 10.00000000000000000 ) ) ;
#5193=CARTESIAN_POINT ( 'NONE',  ( 1.631735293711821022, 4.895207720155140940, 10.00000000000000000 ) ) ;
#5202=CARTESIAN_POINT ( 'NONE',  ( -8.665663522307772482, -5.581295667939712324, 6.857782953271941950E-17 ) ) ;
#5209=CARTESIAN_POINT ( 'NONE',  ( -9.680665087126289592, -7.686621967951973389, 10.00000000000000000 ) ) ;
#5216=CARTESIAN_POINT ( 'NONE',  ( -8.209791827104817585, -6.297951179201753291, 10.00000000000000000 ) ) ;
#5218=CARTESIAN_POINT ( 'NONE',  ( 9.623054350189519823, -9.012277985855606133, 3.747395293195558847E-16 ) ) ;
#5229=CARTESIAN_POINT ( 'NONE',  ( -9.820986981721938847, 1.626514086989861108, 6.857782953271941950E-17 ) ) ;
#5237=EDGE_CURVE ( 'NONE', #4165, #3870, #5432, .T. ) ;
#5238=CARTESIAN_POINT ( 'NONE',  ( -6.777230418910823673, -10.52530689671158548, 10.00000000000000000 ) ) ;
#5243=CARTESIAN_POINT ( 'NONE',  ( -5.962113107391269651, -1.426310550302858582, 3.747395293195558847E-16 ) ) ;
#5248=CARTESIAN_POINT ( 'NONE',  ( 1.124919223378051392, -13.78906249641292270, 10.00000000000000000 ) ) ;
#5259=CARTESIAN_POINT ( 'NONE',  ( 9.246005348854470896, -6.405614325511344909, 6.857782953271941950E-17 ) ) ;
#5265=CARTESIAN_POINT ( 'NONE',  ( -2.196651480121881050, 8.111327970581173830, 10.00000000000000000 ) ) ;
#5276=CARTESIAN_POINT ( 'NONE',  ( -10.03906249502029091, -0.8181230654450249995, 10.00000000000000000 ) ) ;
#5278=CARTESIAN_POINT ( 'NONE',  ( 10.36190401370965475, -8.216093097539266310, 3.747395293195558847E-16 ) ) ;
#5292=CARTESIAN_POINT ( 'NONE',  ( -4.006926059189011902, 5.225193401749456790, 10.00000000000000000 ) ) ;
#5293=CARTESIAN_POINT ( 'NONE',  ( -8.201440678127905670, 5.289679325232165219, 6.857782953271941950E-17 ) ) ;
#5303=CARTESIAN_POINT ( 'NONE',  ( -11.74902089294173813, -3.156991809147611683, 10.00000000000000000 ) ) ;
#5309=CARTESIAN_POINT ( 'NONE',  ( 2.581500635392914411, -6.456130005640034142, 3.747395293195558847E-16 ) ) ;
#5319=CARTESIAN_POINT ( 'NONE',  ( 3.571029491936648093, 3.388293644658559423, 10.00000000000000000 ) ) ;
#5326=CARTESIAN_POINT ( 'NONE',  ( -9.023584016175915323, 3.917288190900554579, 6.857782953271941950E-17 ) ) ;
#5336=CARTESIAN_POINT ( 'NONE',  ( 1.831757423467613277, 7.960349185506228942, 10.00000000000000000 ) ) ;
#5339=DIRECTION ( 'NONE',  ( 4.336808689942017736E-17, 6.938893903907228378E-16, -1.000000000000000000 ) ) ;
#5344=CARTESIAN_POINT ( 'NONE',  ( -6.589974825828277538, 7.038139701356666222, 10.00000000000000000 ) ) ;
#5354=CARTESIAN_POINT ( 'NONE',  ( -1.790740696106538632, -6.394195405909704810, 3.747395293195558847E-16 ) ) ;
#5360=CARTESIAN_POINT ( 'NONE',  ( 1.022653496104248827, 6.171874473422430007, 10.00000000000000000 ) ) ;
#5361=CARTESIAN_POINT ( 'NONE',  ( 10.63538685525200478, -4.008487272325076844, 6.857782953271941950E-17 ) ) ;
#5370=CARTESIAN_POINT ( 'NONE',  ( 13.29800827116429929, 3.099979537169774257, 10.00000000000000000 ) ) ;
#5374=CARTESIAN_POINT ( 'NONE',  ( -0.9167995209625431352, 5.268308710424121521, 3.747395293195558847E-16 ) ) ;
#5386=CARTESIAN_POINT ( 'NONE',  ( 16.50000000000000000, 0.000000000000000000, 3.747395293195558847E-16 ) ) ;
#5387=CARTESIAN_POINT ( 'NONE',  ( -6.451445390047170214, -3.308750875808896819, 6.857782953271941950E-17 ) ) ;
#5391=CARTESIAN_POINT ( 'NONE',  ( 6.563569809674243416, -3.208372544468512721, 10.00000000000000000 ) ) ;
#5394=LINE ( 'NONE', #8086, #2071 ) ;
#5400=CARTESIAN_POINT ( 'NONE',  ( 1.022653496104248827, 6.171874473422430007, 10.00000000000000000 ) ) ;
#5407=CARTESIAN_POINT ( 'NONE',  ( 2.084958754360775934, -3.480815169281481047, 3.747395293195558847E-16 ) ) ;
#5414=CARTESIAN_POINT ( 'NONE',  ( 3.913389251769919586, -3.458713887698555922, 10.00000000000000000 ) ) ;
#5415=CARTESIAN_POINT ( 'NONE',  ( 8.143984375791809782, 3.063465613658396425, 6.857782953271941950E-17 ) ) ;
#5421=CARTESIAN_POINT ( 'NONE',  ( -8.207979594962568015, -13.19054478262514607, 10.00000000000000000 ) ) ;
#5425=CARTESIAN_POINT ( 'NONE',  ( -3.231136241382283725, -5.666136714102345984, 3.747395293195558847E-16 ) ) ;
#5432=LINE ( 'NONE', #4584, #10543 ) ;
#5445=CARTESIAN_POINT ( 'NONE',  ( 3.120778274233608318, -6.257845451232916467, 10.00000000000000000 ) ) ;
#5452=CARTESIAN_POINT ( 'NONE',  ( 10.64229886435067662, -13.41933351754326154, 6.857782953271941950E-17 ) ) ;
#5462=CARTESIAN_POINT ( 'NONE',  ( -3.663109177303993214, -5.348850660921103284, 3.747395293195558847E-16 ) ) ;
#5469=CARTESIAN_POINT ( 'NONE',  ( 2.919619825260425294, -7.400844473264723611, 6.857782953271941950E-17 ) ) ;
#5478=CARTESIAN_POINT ( 'NONE',  ( -6.430932688512554840, -6.885836206078318256, 10.00000000000000000 ) ) ;
#5484=CARTESIAN_POINT ( 'NONE',  ( 7.078846155421574693, 8.354583459611243157, 3.747395293195558847E-16 ) ) ;
#5493=CARTESIAN_POINT ( 'NONE',  ( -1.103316172498963521, -16.73802372459124044, 6.857782953271941950E-17 ) ) ;
#5504=CARTESIAN_POINT ( 'NONE',  ( -15.05755265055531034, -0.4891349978715467950, 3.747395293195558847E-16 ) ) ;
#5505=CARTESIAN_POINT ( 'NONE',  ( -7.040021908109678428, -0.4595208068204874041, 6.857782953271941950E-17 ) ) ;
#5514=CARTESIAN_POINT ( 'NONE',  ( -2.296015608618633852, -6.188270089872266233, 10.00000000000000000 ) ) ;
#5521=CARTESIAN_POINT ( 'NONE',  ( 3.666996827460253350, 4.772409917195344242, 10.00000000000000000 ) ) ;
#5530=CARTESIAN_POINT ( 'NONE',  ( -5.962113107391269651, -1.426310550302858582, 3.747395293195558847E-16 ) ) ;
#5537=CARTESIAN_POINT ( 'NONE',  ( -5.924299593718516554, 3.297400215539475710, 6.857782953271941950E-17 ) ) ;
#5548=CARTESIAN_POINT ( 'NONE',  ( 0.6578947103914143391, -9.792230064638474119, 10.00000000000000000 ) ) ;
#5553=CARTESIAN_POINT ( 'NONE',  ( 8.913847851857145344, -5.129921849437907078, 3.747395293195558847E-16 ) ) ;
#5566=CARTESIAN_POINT ( 'NONE',  ( 10.01890055165174864, -12.63311126014528796, 3.747395293195558847E-16 ) ) ;
#5567=CARTESIAN_POINT ( 'NONE',  ( -5.248573321596925467, 4.168074790661427720, 6.857782953271941950E-17 ) ) ;
#5575=CARTESIAN_POINT ( 'NONE',  ( 0.5697670706242778937, -3.781298318517896551, 10.00000000000000000 ) ) ;
#5581=CARTESIAN_POINT ( 'NONE',  ( 2.529667540517110513, -4.392173529266737653, 10.00000000000000000 ) ) ;
#5590=CARTESIAN_POINT ( 'NONE',  ( -5.541928854458315179, -2.884958602215172085, 3.747395293195558847E-16 ) ) ;
#5594=CARTESIAN_POINT ( 'NONE',  ( -16.06046882360140060, -0.5196555361422392494, 10.00000000000000000 ) ) ;
#5596=CARTESIAN_POINT ( 'NONE',  ( 3.534825977509324257, -7.171832907601985774, 6.857782953271941950E-17 ) ) ;
#5604=CARTESIAN_POINT ( 'NONE',  ( -7.402161455537875412, -5.702533393948235663, 10.00000000000000000 ) ) ;
#5607=CARTESIAN_POINT ( 'NONE',  ( -7.402161455537873636, -5.702533393948970186, 3.747395293195558847E-16 ) ) ;
#5608=EDGE_CURVE ( 'NONE', #7701, #3870, #1507, .T. ) ;
#5620=PLANE ( 'NONE',  #750 ) ;
#5623=CARTESIAN_POINT ( 'NONE',  ( -14.60057116351879714, -4.165219547604622541, 3.747395293195558847E-16 ) ) ;
#5624=CARTESIAN_POINT ( 'NONE',  ( -6.211147023100837217, 2.816369743025007644, 6.857782953271941950E-17 ) ) ;
#5638=CARTESIAN_POINT ( 'NONE',  ( 2.004495162477544223, 5.838205294495796949, 10.00000000000000000 ) ) ;
#5647=CARTESIAN_POINT ( 'NONE',  ( 1.629745903656676820, 14.14889381255350287, 10.00000000000000000 ) ) ;
#5655=CARTESIAN_POINT ( 'NONE',  ( -10.11701526667144257, 11.92482893257633947, 10.00000000000000000 ) ) ;
#5656=CARTESIAN_POINT ( 'NONE',  ( -2.570438583093345386, 5.934334910739564428, 6.857782953271941950E-17 ) ) ;
#5660=CARTESIAN_POINT ( 'NONE',  ( 17.49999999999999645, 0.000000000000000000, 6.857782953271941950E-17 ) ) ;
#5664=CARTESIAN_POINT ( 'NONE',  ( 8.282588618526579793, 7.043362411858248073, 10.00000000000000000 ) ) ;
#5668=CARTESIAN_POINT ( 'NONE',  ( 6.391761267590965190, 8.940137919805573929, 3.747395293195558847E-16 ) ) ;
#5669=CARTESIAN_POINT ( 'NONE',  ( 4.516389116325773223, 1.247036727255508515, 3.747395293195558847E-16 ) ) ;
#5686=CARTESIAN_POINT ( 'NONE',  ( 7.795318149608630343, -14.02504990431079612, 3.747395293195558847E-16 ) ) ;
#5705=CARTESIAN_POINT ( 'NONE',  ( -10.11701526667143725, 11.92482893257633414, 6.857782953271941950E-17 ) ) ;
#5715=CARTESIAN_POINT ( 'NONE',  ( 11.04976219204224996, -11.79656285005915350, 10.00000000000000000 ) ) ;
#5724=CARTESIAN_POINT ( 'NONE',  ( 3.017784444055084947, -16.62017357425736463, 10.00000000000000000 ) ) ;
#5733=CARTESIAN_POINT ( 'NONE',  ( -3.141381368647836236, 10.98006565327106543, 10.00000000000000000 ) ) ;
#5737=CARTESIAN_POINT ( 'NONE',  ( -8.109405675832187299, 8.372220220304370741, 3.747395293195558847E-16 ) ) ;
#5739=( GEOMETRIC_REPRESENTATION_CONTEXT ( 3 ) GLOBAL_UNCERTAINTY_ASSIGNED_CONTEXT ( ( #7317 ) ) GLOBAL_UNIT_ASSIGNED_CONTEXT ( ( #9205, #7487, #8355 ) ) REPRESENTATION_CONTEXT ( 'NONE', 'WORKASPACE' ) );
#5740=CARTESIAN_POINT ( 'NONE',  ( -1.124919223378054722, -13.71093750358708085, 6.857782953271941950E-17 ) ) ;
#5753=CARTESIAN_POINT ( 'NONE',  ( -6.423942855642367000, 13.01866063961475461, 3.747395293195558847E-16 ) ) ;
#5757=CARTESIAN_POINT ( 'NONE',  ( -13.43906451854578954, -9.301052350413227643, 10.00000000000000000 ) ) ;
#5759=CARTESIAN_POINT ( 'NONE',  ( 2.084958754360777711, -3.480815169282206689, 10.00000000000000000 ) ) ;
#5765=CARTESIAN_POINT ( 'NONE',  ( 1.124919223378051392, -13.78906249641291559, 6.857782953271941950E-17 ) ) ;
#5775=CARTESIAN_POINT ( 'NONE',  ( 13.53515989517831919, -0.2218654272303337005, 10.00000000000000000 ) ) ;
#5779=CARTESIAN_POINT ( 'NONE',  ( 14.52660474336492236, -9.366294961249355566, 6.857782953271941950E-17 ) ) ;
#5782=CARTESIAN_POINT ( 'NONE',  ( -5.414455899168761022, -12.47541146649038879, 10.00000000000000000 ) ) ;
#5784=CARTESIAN_POINT ( 'NONE',  ( -14.61026919807147095, 3.159152207411756397, 3.747395293195558847E-16 ) ) ;
#5791=CARTESIAN_POINT ( 'NONE',  ( 7.536008357046525497, 0.2705779428718255719, 10.00000000000000000 ) ) ;
#5794=CARTESIAN_POINT ( 'NONE',  ( -3.909826107003197215, 8.641065831729468627, 10.00000000000000000 ) ) ;
#5795=CARTESIAN_POINT ( 'NONE',  ( 11.20109743375191691, 9.815261043521076090, 6.857782953271941950E-17 ) ) ;
#5805=DIRECTION ( 'NONE',  ( 0.07332096784668425127, 0.9973083954695386444, 3.060346140701604533E-16 ) ) ;
#5808=CARTESIAN_POINT ( 'NONE',  ( -1.035167565893234443, -12.71157708251009133, 3.747395293195558847E-16 ) ) ;
#5812=SHAPE_REPRESENTATION_RELATIONSHIP ( 'NONE' , 'NONE' ,  #7555, #7312 ) ;
#5813=CARTESIAN_POINT ( 'NONE',  ( -11.80455809908110432, -11.41585333555581983, 10.00000000000000000 ) ) ;
#5821=CARTESIAN_POINT ( 'NONE',  ( -14.19814495527598730, 7.008511237308412412, 6.857782953271941950E-17 ) ) ;
#5831=CARTESIAN_POINT ( 'NONE',  ( 13.03626601087043113, 4.193914020169875911, 10.00000000000000000 ) ) ;
#5834=CARTESIAN_POINT ( 'NONE',  ( 17.46093749967478104, -1.431715403549062460, 6.857782953271941950E-17 ) ) ;
#5838=CARTESIAN_POINT ( 'NONE',  ( -3.406233159845097891, 11.94786423299365197, 10.00000000000000000 ) ) ;
#5840=CARTESIAN_POINT ( 'NONE',  ( -11.99326810842395474, 8.590522060507202795, 3.747395293195558847E-16 ) ) ;
#5850=CARTESIAN_POINT ( 'NONE',  ( 4.623190192904714557, -5.402202315098911356, 10.00000000000000000 ) ) ;
#5852=CARTESIAN_POINT ( 'NONE',  ( -4.368568794346924022, -9.638580752213403713, 10.00000000000000000 ) ) ;
#5854=CARTESIAN_POINT ( 'NONE',  ( -13.43906451854462603, -9.301052350413224090, 6.857782953271941950E-17 ) ) ;
#5857=ORIENTED_EDGE ( 'NONE', *, *, #7856, .T. ) ;
#5865=CARTESIAN_POINT ( 'NONE',  ( 7.316052646047088714, -7.060001943526879487, 3.747395293195558847E-16 ) ) ;
#5870=ORIENTED_EDGE ( 'NONE', *, *, #213, .F. ) ;
#5872=CARTESIAN_POINT ( 'NONE',  ( 0.07364157424580704270, -3.751631698233870438, 3.747395293195558847E-16 ) ) ;
#5883=CARTESIAN_POINT ( 'NONE',  ( -5.683926142426733108, 14.39978054689283660, 6.857782953271941950E-17 ) ) ;
#5891=CARTESIAN_POINT ( 'NONE',  ( 2.103398428914359908, -12.69820342197951035, 10.00000000000000000 ) ) ;
#5897=CARTESIAN_POINT ( 'NONE',  ( 5.334478431285540445, 14.15651896542077104, 10.00000000000000000 ) ) ;
#5900=CARTESIAN_POINT ( 'NONE',  ( 10.01890055165174864, -12.63311126014528796, 3.747395293195558847E-16 ) ) ;
#5908=CARTESIAN_POINT ( 'NONE',  ( 3.656769781543558917, 7.172433557890307121, 10.00000000000000000 ) ) ;
#5914=CARTESIAN_POINT ( 'NONE',  ( -8.665663522307777811, -5.581295667939715877, 10.00000000000000000 ) ) ;
#5916=CARTESIAN_POINT ( 'NONE',  ( -11.61414229320030067, -6.453515506896104981, 6.857782953271941950E-17 ) ) ;
#5928=CARTESIAN_POINT ( 'NONE',  ( 3.053028024665286111, -9.450988318041344982, 3.747395293195558847E-16 ) ) ;
#5936=CARTESIAN_POINT ( 'NONE',  ( 4.165359127293308816, 14.58480927028733554, 10.00000000000000000 ) ) ;
#5938=CARTESIAN_POINT ( 'NONE',  ( 7.014224211608840243, -15.49593329755746218, 6.857782953271941950E-17 ) ) ;
#5946=CARTESIAN_POINT ( 'NONE',  ( 12.50121531544688480, -6.953993600215016002, 6.857782953271941950E-17 ) ) ;
#5952=CARTESIAN_POINT ( 'NONE',  ( 10.51453309316909568, -0.3307463982597985686, 10.00000000000000000 ) ) ;
#5959=CARTESIAN_POINT ( 'NONE',  ( 12.50121531544689013, -6.953993600215019555, 10.00000000000000000 ) ) ;
#5961=CARTESIAN_POINT ( 'NONE',  ( 15.00667705184753764, -6.512453894250635145, 3.747395293195558847E-16 ) ) ;
#5970=CARTESIAN_POINT ( 'NONE',  ( -9.960937504979712642, 0.8181230654450121209, 10.00000000000000000 ) ) ;
#5972=CARTESIAN_POINT ( 'NONE',  ( 4.479449988082533807, -13.21383449271837840, 6.857782953271941950E-17 ) ) ;
#5984=CARTESIAN_POINT ( 'NONE',  ( -5.773631947676829412, 9.989728373610901713, 3.747395293195558847E-16 ) ) ;
#5992=CARTESIAN_POINT ( 'NONE',  ( 13.99323099383125069, 4.495563823643928814, 10.00000000000000000 ) ) ;
#6000=CARTESIAN_POINT ( 'NONE',  ( 11.50231346626665285, 1.508968394323198847, 6.857782953271941950E-17 ) ) ;
#6006=CARTESIAN_POINT ( 'NONE',  ( -6.430932688512554840, -6.885836206078318256, 10.00000000000000000 ) ) ;
#6012=CARTESIAN_POINT ( 'NONE',  ( -12.06849956494803600, -5.462025159505909500, 10.00000000000000000 ) ) ;
#6016=CARTESIAN_POINT ( 'NONE',  ( 16.50000000000000000, 0.000000000000000000, 3.747395293195558847E-16 ) ) ;
#6018=ORIENTED_EDGE ( 'NONE', *, *, #5608, .T. ) ;
#6027=CARTESIAN_POINT ( 'NONE',  ( -8.209791827104817585, -6.297951179201753291, 10.00000000000000000 ) ) ;
#6028=CARTESIAN_POINT ( 'NONE',  ( 8.025946968469181542, -7.769110617520081696, 6.857782953271941950E-17 ) ) ;
#6039=CARTESIAN_POINT ( 'NONE',  ( -1.307086582042907619, 11.26718560147321213, 3.747395293195558847E-16 ) ) ;
#6047=CARTESIAN_POINT ( 'NONE',  ( -0.3972327064967878796, 12.29993208790120640, 10.00000000000000000 ) ) ;
#6059=CARTESIAN_POINT ( 'NONE',  ( 5.893263639826756162, 6.717612500731040548, 6.857782953271941950E-17 ) ) ;
#6066=CARTESIAN_POINT ( 'NONE',  ( -11.15100792855599110, -5.055838994807845488, 10.00000000000000000 ) ) ;
#6073=CARTESIAN_POINT ( 'NONE',  ( 8.329772390959204742, 2.373743296044067641, 10.00000000000000000 ) ) ;
#6077=CARTESIAN_POINT ( 'NONE',  ( 13.24268851590353790, -2.403973981684889072, 3.747395293195558847E-16 ) ) ;
#6091=CARTESIAN_POINT ( 'NONE',  ( -4.263796145714478847, -6.152586724582791433, 10.00000000000000000 ) ) ;
#6092=CARTESIAN_POINT ( 'NONE',  ( -9.023584016175915323, 3.917288190900554579, 6.857782953271941950E-17 ) ) ;
#6106=CARTESIAN_POINT ( 'NONE',  ( -2.196651480121880162, 8.111327970581170277, 3.747395293195558847E-16 ) ) ;
#6113=CARTESIAN_POINT ( 'NONE',  ( -13.04979933117209967, -0.2127334381860513379, 10.00000000000000000 ) ) ;
#6123=CARTESIAN_POINT ( 'NONE',  ( -0.1814876354083659327, -10.77628937513454943, 6.857782953271941950E-17 ) ) ;
#6125=MECHANICAL_DESIGN_GEOMETRIC_PRESENTATION_REPRESENTATION('',(#11594),#5739);
#6132=CARTESIAN_POINT ( 'NONE',  ( 1.454091968623351550, 11.13059540125182778, 10.00000000000000000 ) ) ;
#6140=CARTESIAN_POINT ( 'NONE',  ( -5.965338750500730924, 7.524205049158505965, 10.00000000000000000 ) ) ;
#6143=CARTESIAN_POINT ( 'NONE',  ( -11.62103867303406624, 2.700230667072888835, 3.747395293195558847E-16 ) ) ;
#6150=APPLICATION_CONTEXT ( 'automotive_design' ) ;
#6157=CARTESIAN_POINT ( 'NONE',  ( 7.737545192982509867, 9.111483571581276308, 6.857782953271941950E-17 ) ) ;
#6162=ORIENTED_EDGE ( 'NONE', *, *, #5237, .T. ) ;
#6164=CARTESIAN_POINT ( 'NONE',  ( 0.4634152073531427884, 14.27464310366533695, 10.00000000000000000 ) ) ;
#6167=CARTESIAN_POINT ( 'NONE',  ( -2.296015608618632076, -6.188270089871726221, 3.747395293195558847E-16 ) ) ;
#6174=CARTESIAN_POINT ( 'NONE',  ( -9.546882484473293573, 8.373557015401750903, 10.00000000000000000 ) ) ;
#6175=ORIENTED_EDGE ( 'NONE', *, *, #12012, .T. ) ;
#6176=CARTESIAN_POINT ( 'NONE',  ( -2.214925388402925410, 4.996014981202114846, 10.00000000000000000 ) ) ;
#6185=CARTESIAN_POINT ( 'NONE',  ( 9.623984404417814886, 6.889883918979093025, 6.857782953271941950E-17 ) ) ;
#6191=CARTESIAN_POINT ( 'NONE',  ( 7.316052646047090491, -7.060001943526881263, 10.00000000000000000 ) ) ;
#6197=CARTESIAN_POINT ( 'NONE',  ( 7.763517025773944980, -3.069710483245354116, 10.00000000000000000 ) ) ;
#6199=CARTESIAN_POINT ( 'NONE',  ( 4.977139221860116258, 13.21892491369776934, 3.747395293195558847E-16 ) ) ;
#6211=CARTESIAN_POINT ( 'NONE',  ( 9.623984404417814886, 6.889883918979093025, 6.857782953271941950E-17 ) ) ;
#6219=CARTESIAN_POINT ( 'NONE',  ( -10.73274959028002229, -5.974010873319484105, 10.00000000000000000 ) ) ;
#6225=CARTESIAN_POINT ( 'NONE',  ( -6.012500708481076650, 0.06204199954272016787, 3.747395293195558847E-16 ) ) ;
#6232=CARTESIAN_POINT ( 'NONE',  ( 0.8073695008816145213, 5.181225205791319510, 10.00000000000000000 ) ) ;
#6242=CARTESIAN_POINT ( 'NONE',  ( 3.343943643650757913, -10.41127694127634129, 6.857782953271941950E-17 ) ) ;
#6249=CARTESIAN_POINT ( 'NONE',  ( -4.158472309566741743, 3.840014155104743754, 10.00000000000000000 ) ) ;
#6256=CARTESIAN_POINT ( 'NONE',  ( -9.977213461302319786, -1.645879626164742593, 10.00000000000000000 ) ) ;
#6264=CARTESIAN_POINT ( 'NONE',  ( 3.194803811556592876, -2.743189786380903161, 3.747395293195558847E-16 ) ) ;
#6272=CARTESIAN_POINT ( 'NONE',  ( -2.100379401128186441, -7.348625593045292170, 10.00000000000000000 ) ) ;
#6273=CARTESIAN_POINT ( 'NONE',  ( 10.54603994011982415, 5.199563424939647405, 6.857782953271941950E-17 ) ) ;
#6274=MECHANICAL_DESIGN_GEOMETRIC_PRESENTATION_REPRESENTATION('',(#4124),#10963);
#6283=CARTESIAN_POINT ( 'NONE',  ( -11.08238827499401680, -10.71925978067563001, 10.00000000000000000 ) ) ;
#6284=EDGE_CURVE ( 'NONE', #3450, #7701, #7797, .T. ) ;
#6290=CARTESIAN_POINT ( 'NONE',  ( -4.491015865170908228, 3.510096388331549910, 3.747395293195558847E-16 ) ) ;
#6307=CARTESIAN_POINT ( 'NONE',  ( 0.0002901587068756704066, -4.749354241797638210, 6.857782953271941950E-17 ) ) ;
#6314=CARTESIAN_POINT ( 'NONE',  ( -3.231136241382285501, -5.666136714101813965, 10.00000000000000000 ) ) ;
#6324=CARTESIAN_POINT ( 'NONE',  ( -11.80455809908225717, -11.41585333555581627, 6.857782953271941950E-17 ) ) ;
#6331=CARTESIAN_POINT ( 'NONE',  ( 3.678979105947487671, -2.215585777442455662, 3.747395293195558847E-16 ) ) ;
#6340=CARTESIAN_POINT ( 'NONE',  ( 7.763517025772753044, -3.069710483245351451, 6.857782953271941950E-17 ) ) ;
#6347=CARTESIAN_POINT ( 'NONE',  ( -14.85975435031504865, 1.953672781916663936, 10.00000000000000000 ) ) ;
#6350=CARTESIAN_POINT ( 'NONE',  ( 3.120778274233606098, -6.257845451233481349, 3.747395293195558847E-16 ) ) ;
#6356=CARTESIAN_POINT ( 'NONE',  ( 2.084958754360777711, -3.480815169282206689, 10.00000000000000000 ) ) ;
#6357=EDGE_CURVE ( 'NONE', #1474, #3450, #8901, .T. ) ;
#6363=CARTESIAN_POINT ( 'NONE',  ( 5.267519402444978738, 2.381954139586884622, 6.857782953271941950E-17 ) ) ;
#6371=CARTESIAN_POINT ( 'NONE',  ( 2.467392210070201486, 7.745125807189176648, 10.00000000000000000 ) ) ;
#6378=CARTESIAN_POINT ( 'NONE',  ( -3.542987847618590536, 5.503081486278161627, 10.00000000000000000 ) ) ;
#6385=CARTESIAN_POINT ( 'NONE',  ( 7.536008357046521944, 0.2705779428718260160, 3.747395293195558847E-16 ) ) ;
#6390=CARTESIAN_POINT ( 'NONE',  ( -14.19814495527487352, 7.008511237308415964, 10.00000000000000000 ) ) ;
#6391=CARTESIAN_POINT ( 'NONE',  ( -5.248573321596925467, 4.168074790661427720, 6.857782953271941950E-17 ) ) ;
#6398=CARTESIAN_POINT ( 'NONE',  ( 11.62709622633371076, -6.461356448465072511, 10.00000000000000000 ) ) ;
#6401=CARTESIAN_POINT ( 'NONE',  ( -1.719633853164446613, -9.543036404944416518, 3.747395293195558847E-16 ) ) ;
#6418=CARTESIAN_POINT ( 'NONE',  ( 4.698850784960272087, -6.565226861933591174, 6.857782953271941950E-17 ) ) ;
#6427=CARTESIAN_POINT ( 'NONE',  ( 4.140589500486091090, -5.731468560951012314, 10.00000000000000000 ) ) ;
#6436=CARTESIAN_POINT ( 'NONE',  ( -0.5113267480521390684, 6.289062763288780999, 10.00000000000000000 ) ) ;
#6442=CARTESIAN_POINT ( 'NONE',  ( -2.214925388403154116, 4.996014981202573146, 3.747395293195558847E-16 ) ) ;
#6450=CARTESIAN_POINT ( 'NONE',  ( 6.689389171169558779, -4.795626085247174153, 6.857782953271941950E-17 ) ) ;
#6458=CARTESIAN_POINT ( 'NONE',  ( -1.515734900794040829, 8.225284064336937817, 10.00000000000000000 ) ) ;
#6462=CARTESIAN_POINT ( 'NONE',  ( 3.053028024665286111, -9.450988318041344982, 3.747395293195558847E-16 ) ) ;
#6463=CARTESIAN_POINT ( 'NONE',  ( 4.340769014460001962, -0.9713985772308075806, 3.747395293195558847E-16 ) ) ;
#6477=CARTESIAN_POINT ( 'NONE',  ( 13.54728169684850059, 0.8932250400879224728, 3.747395293195558847E-16 ) ) ;
#6478=CARTESIAN_POINT ( 'NONE',  ( -1.032305814202111760, 6.265050879046235366, 6.857782953271941950E-17 ) ) ;
#6487=CARTESIAN_POINT ( 'NONE',  ( 0.07364157424580680678, -3.751631698233684364, 10.00000000000000000 ) ) ;
#6494=CARTESIAN_POINT ( 'NONE',  ( -3.791520748785365491, -16.26028641251512497, 6.857782953271941950E-17 ) ) ;
#6504=CARTESIAN_POINT ( 'NONE',  ( -3.432991321284826647, 4.402131891631369420, 3.747395293195558847E-16 ) ) ;
#6509=CARTESIAN_POINT ( 'NONE',  ( -11.80455809908110432, -11.41585333555581983, 10.00000000000000000 ) ) ;
#6512=CARTESIAN_POINT ( 'NONE',  ( 6.396238541184324333, 6.183590428399971195, 6.857782953271941950E-17 ) ) ;
#6522=CARTESIAN_POINT ( 'NONE',  ( 10.00611923916671309, -2.842981073525690405, 10.00000000000000000 ) ) ;
#6525=CARTESIAN_POINT ( 'NONE',  ( -1.307086582042907619, 11.26718560147321213, 3.747395293195558847E-16 ) ) ;
#6526=CARTESIAN_POINT ( 'NONE',  ( 3.006682760306612856, 4.002877712838976976, 3.747395293195558847E-16 ) ) ;
#6539=CARTESIAN_POINT ( 'NONE',  ( 7.972781652389871354, 11.51689705412852405, 3.747395293195558847E-16 ) ) ;
#6540=CARTESIAN_POINT ( 'NONE',  ( 1.737537816361722331, -4.672682311025833535, 6.857782953271941950E-17 ) ) ;
#6553=CARTESIAN_POINT ( 'NONE',  ( -7.014275365397510065, 0.1192422097806477982, 10.00000000000000000 ) ) ;
#6561=CARTESIAN_POINT ( 'NONE',  ( 0.4634152073531427884, 14.27464310366533695, 10.00000000000000000 ) ) ;
#6566=CARTESIAN_POINT ( 'NONE',  ( 0.2749788638910979355, -16.81181333738675931, 10.00000000000000000 ) ) ;
#6568=CARTESIAN_POINT ( 'NONE',  ( -7.014275365397503847, 0.1192422097806469378, 6.857782953271941950E-17 ) ) ;
#6576=CARTESIAN_POINT ( 'NONE',  ( -6.925491926712309620, 5.292860106065908177, 10.00000000000000000 ) ) ;
#6581=CARTESIAN_POINT ( 'NONE',  ( 8.429646098664187903, -5.822225404888638600, 3.747395293195558847E-16 ) ) ;
#6584=VERTEX_POINT ( 'NONE', #3818 ) ;
#6594=CARTESIAN_POINT ( 'NONE',  ( -15.00596061316373842, -1.728743269517114323, 3.747395293195558847E-16 ) ) ;
#6595=B_SPLINE_SURFACE_WITH_KNOTS ( 'NONE', 1, 3, ( 
 ( #6016, #10669, #9743, #4922, #5961, #9568, #9688, #1361, #5900, #5038, #1181, #6748, #1252, #11410, #4184, #10427, #8774, #4856, #4003, #11466, #5095, #3087, #4984, #1123, #9507, #8719, #8662, #4058, #5784, #7911, #7789, #5840, #379, #4120, #3031, #262, #7853, #10486, #11642, #2101, #6689, #1542, #6199, #11763, #560, #9924, #4294, #9810, #8095, #8028, #1483, #7040, #2340, #6077, #7101, #4239, #10851, #5278, #5218, #11822, #7157, #1424, #3388, #2460, #9012, #628, #3447, #4358, #3261, #6980, #10725, #2401, #10791, #5157, #8895, #500, #7965, #11698, #3320, #6143, #9871, #8951, #11299, #10312, #5737, #3713, #1930, #8431, #7433, #6525, #1746, #955, #10197, #11183, #8303, #5668, #5484, #2733, #31, #9220, #91, #9282, #10375, #2914, #6637, #897, #7499, #5553, #6581, #1996, #1875, #9399, #4632, #6462, #2797, #12027, #4812, #6401, #4756, #838, #12086, #10260, #9462, #5607, #4693, #4574, #3651, #9339, #8363, #3779, #7368, #1079, #11243, #1814, #1024, #3837, #7559, #10127, #2858, #8549, #8493, #146, #3891, #7611, #2670, #11112, #1617, #9135, #8216, #692, #12009, #3690, #1725, #813, #6385, #10238, #4554, #9260, #7348, #8284, #10174, #1790, #1855, #2651, #7226, #8346, #3457, #2597, #880, #5354, #7165, #10054, #5462, #9083, #11093, #7413, #5590, #2708, #5530, #8100, #4425, #4614, #12065, #8158, #3632, #9991, #936, #6504, #11159, #6442, #10976, #9190, #2774, #749, #9321, #11828, #11882, #10910, #3514, #2528, #4483, #6331, #6264, #5407, #1672, #11943, #3575, #7287 ),
 ( #11039, #10109, #9442, #8529, #3755, #2960, #73, #5715, #10296, #7660, #7477, #4738, #2035, #11222, #2094, #11282, #252, #4913, #8651, #2896, #9500, #7538, #8588, #3996, #3871, #185, #6619, #8475, #4793, #1913, #6797, #8406, #6740, #2838, #1973, #1062, #7722, #127, #6679, #6561, #5647, #7594, #10352, #11335, #9378, #11458, #10418, #3817, #3023, #5831, #9561, #5, #5775, #1173, #11401, #10477, #1114, #3078, #10533, #4847, #3935, #2151, #999, #5891, #9623, #4672, #8014, #11688, #9862, #8887, #11514, #7775, #5209, #4284, #6066, #8942, #6970, #9797, #11633, #3376, #1415, #2391, #491, #5149, #3306, #7090, #7902, #369, #1473, #8711, #7843, #6132, #10600, #312, #3200, #10714, #2214, #4229, #550, #10841, #7956, #10779, #1240, #5952, #11753, #2450, #6857, #7030, #3134, #6191, #4975, #4049, #9679, #4109, #2330, #1295, #2273, #5029, #8765, #11580, #6917, #10660, #6006, #9735, #1351, #5084, #8827, #430, #4175, #3250, #8143, #9120, #10037, #2637, #1600, #7394, #11994, #9175, #7331, #5265, #10092, #9916, #4538, #5336, #6371, #1531, #4349, #12052, #617, #11137, #731, #794, #3618, #2580, #677, #1711, #8083, #4599, #5391, #9977, #4466, #11811, #6427, #5445, #9001, #8267, #8202, #11928, #3558, #7270, #5514, #6314, #3439, #10156, #7149, #10898, #3673, #10959, #11079, #1773, #2512, #9069, #11024, #2692, #9245, #1659, #6249, #865, #8330, #2755, #4408, #11868, #3498, #7210, #10337, #10225, #1841, #10460, #12111, #7523, #6604, #11208, #10402, #5759, #3916, #5575, #6663, #6487 ) ),
 .UNSPECIFIED., .F., .F., .F.,
 ( 2, 2 ),
 ( 4, 2, 2, 2, 2, 2, 2, 2, 2, 2, 2, 2, 2, 2, 2, 2, 2, 2, 2, 2, 2, 2, 2, 2, 2, 2, 2, 2, 2, 2, 2, 2, 2, 2, 2, 2, 2, 2, 2, 2, 2, 2, 2, 2, 2, 2, 2, 2, 2, 2, 2, 2, 2, 2, 2, 2, 2, 2, 2, 2, 2, 2, 2, 2, 2, 2, 2, 2, 2, 2, 2, 2, 2, 2, 2, 2, 2, 2, 2, 2, 2, 2, 2, 2, 2, 2, 2, 2, 2, 2, 2, 2, 2, 2, 2, 2, 2, 2, 2, 2, 2, 2, 2, 4 ),
 ( 0.4999999999999998890, 0.9545454545454546968 ),
 ( 0.000000000000000000, 0.007812500000000000000, 0.01562500000000000000, 0.02343750000000000000, 0.03125000000000000000, 0.03906250000000000000, 0.04687500000000000000, 0.05468750000000000000, 0.06250000000000000000, 0.07031250000000000000, 0.07812500000000000000, 0.08593750000000000000, 0.09375000000000000000, 0.1015625000000000000, 0.1093750000000000000, 0.1171875000000000000, 0.1250000000000000000, 0.1328125000000000000, 0.1406250000000000000, 0.1484375000000000000, 0.1562500000000000000, 0.1640625000000000000, 0.1718750000000000000, 0.1796875000000000000, 0.1875000000000000000, 0.1953125000000000000, 0.2031250000000000000, 0.2109375000000000000, 0.2187500000000000000, 0.2265625000000000000, 0.2343750000000000000, 0.2421875000000000000, 0.2500000000000000000, 0.2578125000000000000, 0.2656250000000000000, 0.2734375000000000000, 0.2812500000000000000, 0.2890625000000000000, 0.2968750000000000000, 0.3046875000000000000, 0.3125000000000000000, 0.3203125000000000000, 0.3281250000000000000, 0.3359375000000000000, 0.3437500000000000000, 0.3515625000000000000, 0.3593750000000000000, 0.3671875000000000000, 0.3750000000000000000, 0.3828125000000000000, 0.3906250000000000000, 0.3984375000000000000, 0.4062500000000000000, 0.4140625000000000000, 0.4218750000000000000, 0.4296875000000000000, 0.4375000000000000000, 0.4453125000000000000, 0.4531250000000000000, 0.4609375000000000000, 0.4687500000000000000, 0.4765625000000000000, 0.4843750000000000000, 0.4921875000000000000, 0.5000000000000000000, 0.5078125000000000000, 0.5156250000000000000, 0.5234375000000000000, 0.5312500000000000000, 0.5390625000000000000, 0.5468750000000000000, 0.5546875000000000000, 0.5625000000000000000, 0.5703125000000000000, 0.5781250000000000000, 0.5859375000000000000, 0.5937500000000000000, 0.6015625000000000000, 0.6093750000000000000, 0.6171875000000000000, 0.6250000000000000000, 0.6328125000000000000, 0.6406250000000000000, 0.6484375000000000000, 0.6562500000000000000, 0.6640625000000000000, 0.6718750000000000000, 0.6796875000000000000, 0.6875000000000000000, 0.6953125000000000000, 0.7031250000000000000, 0.7109375000000000000, 0.7187500000000000000, 0.7265625000000000000, 0.7343750000000000000, 0.7421875000000000000, 0.7500000000000000000, 0.7656250000000000000, 0.7812500000000000000, 0.7968750000000000000, 0.8125000000000000000, 0.8281250000000000000, 0.8437500000000000000, 0.8499999999999999778 ),
 .UNSPECIFIED. ) ;
#6604=CARTESIAN_POINT ( 'NONE',  ( 4.340769014460005515, -0.9713985772308084687, 10.00000000000000000 ) ) ;
#6610=CARTESIAN_POINT ( 'NONE',  ( 1.748316258820581170, 15.14524454193558611, 6.857782953271941950E-17 ) ) ;
#6615=EDGE_LOOP ( 'NONE', ( #6667, #2633, #12107, #109 ) ) ;
#6619=CARTESIAN_POINT ( 'NONE',  ( -15.05755265055531389, -0.4891349978715465729, 10.00000000000000000 ) ) ;
#6634=CARTESIAN_POINT ( 'NONE',  ( 3.053028024665676021, -9.450988318042126579, 10.00000000000000000 ) ) ;
#6637=CARTESIAN_POINT ( 'NONE',  ( 10.41236255589546822, -1.188820951657898473, 3.747395293195558847E-16 ) ) ;
#6654=CARTESIAN_POINT ( 'NONE',  ( -1.036640877615904843, -15.73686152240404468, 3.747395293195558847E-16 ) ) ;
#6663=CARTESIAN_POINT ( 'NONE',  ( 0.3190826481552657135, -3.778307095988849618, 10.00000000000000000 ) ) ;
#6667=ORIENTED_EDGE ( 'NONE', *, *, #6898, .F. ) ;
#6670=CARTESIAN_POINT ( 'NONE',  ( -7.159234172427924925, 10.34564589702410942, 6.857782953271941950E-17 ) ) ;
#6679=CARTESIAN_POINT ( 'NONE',  ( -1.872083171988683015, 14.23747171912756393, 10.00000000000000000 ) ) ;
#6686=CARTESIAN_POINT ( 'NONE',  ( -9.783806739528735363, -9.162509837619124298, 10.00000000000000000 ) ) ;
#6689=CARTESIAN_POINT ( 'NONE',  ( 1.629745903656676376, 14.14889381255349932, 3.747395293195558847E-16 ) ) ;
#6697=CARTESIAN_POINT ( 'NONE',  ( 6.723006375386864519, 3.907299473125435796, 10.00000000000000000 ) ) ;
#6701=CARTESIAN_POINT ( 'NONE',  ( 7.252227276002106038, 5.017415995114419047, 10.00000000000000000 ) ) ;
#6704=CARTESIAN_POINT ( 'NONE',  ( -10.85385039129052842, -12.37615246896657339, 6.857782953271941950E-17 ) ) ;
#6716=CARTESIAN_POINT ( 'NONE',  ( 11.72652038055309731, 7.297668919379284524, 3.747395293195558847E-16 ) ) ;
#6732=CARTESIAN_POINT ( 'NONE',  ( 5.564773995946417529, -12.83798980516507626, 6.857782953271941950E-17 ) ) ;
#6740=CARTESIAN_POINT ( 'NONE',  ( -11.21689850596896676, 9.520844388990630236, 10.00000000000000000 ) ) ;
#6746=CARTESIAN_POINT ( 'NONE',  ( 6.986659217179110648, 9.748146710219847577, 10.00000000000000000 ) ) ;
#6748=CARTESIAN_POINT ( 'NONE',  ( 4.123629756449401107, -15.38522696314584515, 3.747395293195558847E-16 ) ) ;
#6757=CARTESIAN_POINT ( 'NONE',  ( -5.962113107391272315, -1.426310550302921865, 10.00000000000000000 ) ) ;
#6760=CARTESIAN_POINT ( 'NONE',  ( 8.527474615971327054, 0.9793716136081388468, 10.00000000000000000 ) ) ;
#6761=CARTESIAN_POINT ( 'NONE',  ( -9.080917052262540423, 12.68274194616037320, 6.857782953271941950E-17 ) ) ;
#6769=CARTESIAN_POINT ( 'NONE',  ( 13.68367311611256909, -8.822018488634764566, 10.00000000000000000 ) ) ;
#6772=CARTESIAN_POINT ( 'NONE',  ( 8.800885721068835821, 6.316044917328127895, 3.747395293195558847E-16 ) ) ;
#6777=CARTESIAN_POINT ( 'NONE',  ( -5.101271054653082615, -15.85638610327791476, 10.00000000000000000 ) ) ;
#6779=CARTESIAN_POINT ( 'NONE',  ( 4.382127860174850120, -16.35473703246190524, 6.857782953271941950E-17 ) ) ;
#6786=CARTESIAN_POINT ( 'NONE',  ( -6.864300873105353418, 13.92024697337931549, 6.857782953271941950E-17 ) ) ;
#6797=CARTESIAN_POINT ( 'NONE',  ( -13.29946171776686903, 6.562258890817373569, 10.00000000000000000 ) ) ;
#6803=CARTESIAN_POINT ( 'NONE',  ( 4.165359127293308816, 14.58480927028733554, 10.00000000000000000 ) ) ;
#6811=ORIENTED_EDGE ( 'NONE', *, *, #6357, .T. ) ;
#6813=CARTESIAN_POINT ( 'NONE',  ( 7.527773320476329744, 0.8933511214756656438, 10.00000000000000000 ) ) ;
#6815=CARTESIAN_POINT ( 'NONE',  ( 0.7062845326068618590, -10.79445016380499212, 10.00000000000000000 ) ) ;
#6817=CARTESIAN_POINT ( 'NONE',  ( 4.165359127293307040, 14.58480927028732843, 6.857782953271941950E-17 ) ) ;
#6824=CARTESIAN_POINT ( 'NONE',  ( 12.88139461472802516, -9.891864711285373701, 10.00000000000000000 ) ) ;
#6828=CARTESIAN_POINT ( 'NONE',  ( 4.583115687978880359, -8.898851689028539624, 3.747395293195558847E-16 ) ) ;
#6836=CARTESIAN_POINT ( 'NONE',  ( -9.080917052262543976, 12.68274194616037853, 10.00000000000000000 ) ) ;
#6848=CARTESIAN_POINT ( 'NONE',  ( -14.76245309360481706, 5.834016798581969532, 6.857782953271941950E-17 ) ) ;
#6857=CARTESIAN_POINT ( 'NONE',  ( 9.701579622838506722, -3.641351606116563389, 10.00000000000000000 ) ) ;
#6859=CLOSED_SHELL ( 'NONE', ( #7119, #746, #4332, #7556, #4826, #11593 ) ) ;
#6863=CARTESIAN_POINT ( 'NONE',  ( -12.91830213043054698, -2.344901317288422327, 10.00000000000000000 ) ) ;
#6874=CARTESIAN_POINT ( 'NONE',  ( 2.467392210070201486, 7.745125807189176648, 10.00000000000000000 ) ) ;
#6879=CARTESIAN_POINT ( 'NONE',  ( 11.37845468071832222, 2.456417158213071161, 10.00000000000000000 ) ) ;
#6881=CARTESIAN_POINT ( 'NONE',  ( -16.06046882360139350, -0.5196555361422402486, 6.857782953271941950E-17 ) ) ;
#6894=CARTESIAN_POINT ( 'NONE',  ( -8.984113827416486231, -1.502549133976348372, 3.747395293195558847E-16 ) ) ;
#6898=EDGE_CURVE ( 'NONE', #1562, #6584, #5394, .T. ) ;
#6900=CARTESIAN_POINT ( 'NONE',  ( 7.619603487155713673, -11.82824555707897218, 10.00000000000000000 ) ) ;
#6910=CARTESIAN_POINT ( 'NONE',  ( 6.986659217179107095, 9.748146710219840472, 6.857782953271941950E-17 ) ) ;
#6917=CARTESIAN_POINT ( 'NONE',  ( -4.622662292628551661, -8.344572748942844953, 10.00000000000000000 ) ) ;
#6923=CARTESIAN_POINT ( 'NONE',  ( 14.27634331491212549, 3.322769473269123974, 10.00000000000000000 ) ) ;
#6933=CARTESIAN_POINT ( 'NONE',  ( -5.125696908148163367, -9.212757455310160992, 10.00000000000000000 ) ) ;
#6935=CARTESIAN_POINT ( 'NONE',  ( -15.85416723795448846, 2.087521067385502693, 6.857782953271941950E-17 ) ) ;
#6942=CARTESIAN_POINT ( 'NONE',  ( 6.600721363681033793, -14.58171973507987751, 10.00000000000000000 ) ) ;
#6946=CARTESIAN_POINT ( 'NONE',  ( -6.597323627731391582, 9.514359934151556786, 3.747395293195558847E-16 ) ) ;
#6953=CARTESIAN_POINT ( 'NONE',  ( -10.47176928358605075, -8.303818807687077808, 10.00000000000000000 ) ) ;
#6963=CARTESIAN_POINT ( 'NONE',  ( 10.54603994011982415, 5.199563424939647405, 6.857782953271941950E-17 ) ) ;
#6970=CARTESIAN_POINT ( 'NONE',  ( -11.92955594661033558, -2.174140050202246766, 10.00000000000000000 ) ) ;
#6973=SURFACE_STYLE_USAGE ( .BOTH. , #1355 ) ;
#6977=CARTESIAN_POINT ( 'NONE',  ( -2.433178163897189883, 9.086443520544605690, 10.00000000000000000 ) ) ;
#6980=CARTESIAN_POINT ( 'NONE',  ( -6.777230418910821896, -10.52530689671158193, 3.747395293195558847E-16 ) ) ;
#6991=CARTESIAN_POINT ( 'NONE',  ( -6.825012239887744414, 1.243808647927287403, 10.00000000000000000 ) ) ;
#6992=CARTESIAN_POINT ( 'NONE',  ( -10.03906249502028558, -0.8181230654450031281, 6.857782953271941950E-17 ) ) ;
#7002=CARTESIAN_POINT ( 'NONE',  ( -8.111627617515257072, 3.498804908652022316, 3.747395293195558847E-16 ) ) ;
#7010=CARTESIAN_POINT ( 'NONE',  ( 5.564773995946421969, -12.83798980516408683, 10.00000000000000000 ) ) ;
#7023=CARTESIAN_POINT ( 'NONE',  ( 2.469054641153893837, -10.61194774715159284, 6.857782953271941950E-17 ) ) ;
#7030=CARTESIAN_POINT ( 'NONE',  ( 8.913847851856345983, -5.129921849437908854, 10.00000000000000000 ) ) ;
#7038=CARTESIAN_POINT ( 'NONE',  ( -0.8869411547437835441, -7.669649013129178350, 10.00000000000000000 ) ) ;
#7040=CARTESIAN_POINT ( 'NONE',  ( 13.54728169684850059, 0.8932250400879224728, 3.747395293195558847E-16 ) ) ;
#7045=DIRECTION ( 'NONE',  ( 3.469446951953614189E-16, 0.000000000000000000, 1.000000000000000000 ) ) ;
#7052=CARTESIAN_POINT ( 'NONE',  ( -7.014275365397510065, 0.1192422097806477982, 10.00000000000000000 ) ) ;
#7053=CARTESIAN_POINT ( 'NONE',  ( 0.6097887191948974106, 9.229167205757265791, 6.857782953271941950E-17 ) ) ;
#7054=FILL_AREA_STYLE_COLOUR ( '', #11204 ) ;
#7061=CARTESIAN_POINT ( 'NONE',  ( -9.045553118584756191, -8.482981269325438944, 10.00000000000000000 ) ) ;
#7066=CARTESIAN_POINT ( 'NONE',  ( -3.516813791735896810, 7.717845097288992484, 3.747395293195558847E-16 ) ) ;
#7071=CARTESIAN_POINT ( 'NONE',  ( -12.59589084681761229, 2.937805917057824789, 10.00000000000000000 ) ) ;
#7082=CARTESIAN_POINT ( 'NONE',  ( -4.368568794346921358, -9.638580752213396607, 6.857782953271941950E-17 ) ) ;
#7086=CARTESIAN_POINT ( 'NONE',  ( 0.07364157424580680678, -3.751631698233684364, 10.00000000000000000 ) ) ;
#7090=CARTESIAN_POINT ( 'NONE',  ( -6.597323627732286866, 9.514359934152452070, 10.00000000000000000 ) ) ;
#7098=CARTESIAN_POINT ( 'NONE',  ( -7.708066421255711731, 5.920849505456871498, 10.00000000000000000 ) ) ;
#7101=CARTESIAN_POINT ( 'NONE',  ( 12.96212312671852551, -3.473279994529273829, 3.747395293195558847E-16 ) ) ;
#7115=CARTESIAN_POINT ( 'NONE',  ( 9.774996403550728630, -5.644905071530503804, 6.857782953271941950E-17 ) ) ;
#7119=ADVANCED_FACE ( 'NONE', ( #11322 ), #4659, .T. ) ;
#7123=CARTESIAN_POINT ( 'NONE',  ( -1.035167565893234443, -12.71157708251009488, 10.00000000000000000 ) ) ;
#7127=CARTESIAN_POINT ( 'NONE',  ( 1.482756436301464920, -6.713508106970949463, 3.747395293195558847E-16 ) ) ;
#7134=CARTESIAN_POINT ( 'NONE',  ( -4.491015865170432164, 3.510096388331073403, 10.00000000000000000 ) ) ;
#7143=CARTESIAN_POINT ( 'NONE',  ( -9.650762677556027569, -3.270672451565358685, 6.857782953271941950E-17 ) ) ;
#7149=CARTESIAN_POINT ( 'NONE',  ( -4.763935748647996959, -4.221771024092342728, 10.00000000000000000 ) ) ;
#7155=CARTESIAN_POINT ( 'NONE',  ( 7.449730884303676248, -3.679036338562946096, 10.00000000000000000 ) ) ;
#7157=CARTESIAN_POINT ( 'NONE',  ( 7.081399987883180813, -10.98142027556026612, 3.747395293195558847E-16 ) ) ;
#7165=CARTESIAN_POINT ( 'NONE',  ( -2.296015608618632076, -6.188270089871726221, 3.747395293195558847E-16 ) ) ;
#7173=CARTESIAN_POINT ( 'NONE',  ( -0.5113267480521390684, 6.289062763288780999, 10.00000000000000000 ) ) ;
#7175=CARTESIAN_POINT ( 'NONE',  ( 11.37845468071831512, 2.456417158213069829, 6.857782953271941950E-17 ) ) ;
#7179=EDGE_LOOP ( 'NONE', ( #2600, #6811, #809, #3440 ) ) ;
#7181=CARTESIAN_POINT ( 'NONE',  ( -11.62103867303406979, 2.700230667072889279, 10.00000000000000000 ) ) ;
#7186=CARTESIAN_POINT ( 'NONE',  ( -5.541928854458315179, -2.884958602215172085, 3.747395293195558847E-16 ) ) ;
#7202=CARTESIAN_POINT ( 'NONE',  ( -6.829322889802579510, -2.192323464439260849, 6.857782953271941950E-17 ) ) ;
#7210=CARTESIAN_POINT ( 'NONE',  ( 0.8073695008816145213, 5.181225205791319510, 10.00000000000000000 ) ) ;
#7218=CARTESIAN_POINT ( 'NONE',  ( 8.539395351299297943, 0.2748098766782894331, 10.00000000000000000 ) ) ;
#7226=CARTESIAN_POINT ( 'NONE',  ( 2.581500635392914411, -6.456130005640034142, 3.747395293195558847E-16 ) ) ;
#7232=CARTESIAN_POINT ( 'NONE',  ( -2.061894914253513456, 6.087690860853038899, 10.00000000000000000 ) ) ;
#7233=CARTESIAN_POINT ( 'NONE',  ( 5.508953106497944674, 1.454581011951804559, 6.857782953271941950E-17 ) ) ;
#7242=CARTESIAN_POINT ( 'NONE',  ( -5.008276813248565773, -11.55791719732261669, 10.00000000000000000 ) ) ;
#7247=CARTESIAN_POINT ( 'NONE',  ( -0.1586286459269546645, 8.284426055182338544, 3.747395293195558847E-16 ) ) ;
#7261=CARTESIAN_POINT ( 'NONE',  ( -3.764233030011069125, -6.516208816467297105, 6.857782953271941950E-17 ) ) ;
#7270=CARTESIAN_POINT ( 'NONE',  ( -1.790740696106539520, -6.394195405909708363, 10.00000000000000000 ) ) ;
#7279=CARTESIAN_POINT ( 'NONE',  ( -6.661525743073271499, 1.789546221321743458, 10.00000000000000000 ) ) ;
#7287=CARTESIAN_POINT ( 'NONE',  ( 0.07364157424580704270, -3.751631698233870438, 3.747395293195558847E-16 ) ) ;
#7293=CARTESIAN_POINT ( 'NONE',  ( 14.52660474336370200, -9.366294961249359119, 10.00000000000000000 ) ) ;
#7294=CARTESIAN_POINT ( 'NONE',  ( 8.329772390959197637, 2.373743296044066309, 6.857782953271941950E-17 ) ) ;
#7300=CARTESIAN_POINT ( 'NONE',  ( -6.423942855642368777, 13.01866063961585951, 10.00000000000000000 ) ) ;
#7312=ADVANCED_BREP_SHAPE_REPRESENTATION ( '', ( #4621, #8474 ), #10565 ) ;
#7317=UNCERTAINTY_MEASURE_WITH_UNIT (LENGTH_MEASURE( 1.000000000000000082E-05 ), #9205, 'distance_accuracy_value', 'NONE');
#7321=CARTESIAN_POINT ( 'NONE',  ( 5.508953106497944674, 1.454581011951804559, 6.857782953271941950E-17 ) ) ;
#7331=CARTESIAN_POINT ( 'NONE',  ( -3.516813791735897254, 7.717845097288996037, 10.00000000000000000 ) ) ;
#7339=CARTESIAN_POINT ( 'NONE',  ( -5.924299593718521884, 3.297400215539481039, 10.00000000000000000 ) ) ;
#7348=CARTESIAN_POINT ( 'NONE',  ( 6.563569809674826061, -3.208372544468511833, 3.747395293195558847E-16 ) ) ;
#7355=CARTESIAN_POINT ( 'NONE',  ( 13.67726327739690184, -10.50289975150004018, 10.00000000000000000 ) ) ;
#7357=CARTESIAN_POINT ( 'NONE',  ( 7.605204090343169909, 4.385345779697310320, 6.857782953271941950E-17 ) ) ;
#7365=CARTESIAN_POINT ( 'NONE',  ( -2.196651480121881050, 8.111327970581173830, 10.00000000000000000 ) ) ;
#7368=CARTESIAN_POINT ( 'NONE',  ( -8.834572391846261752, 1.442725564903823532, 3.747395293195558847E-16 ) ) ;
#7383=CARTESIAN_POINT ( 'NONE',  ( -8.207979594962566239, -13.19054478262514252, 3.747395293195558847E-16 ) ) ;
#7384=CARTESIAN_POINT ( 'NONE',  ( 1.018538006779708738, -7.771884277300779686, 6.857782953271941950E-17 ) ) ;
#7394=CARTESIAN_POINT ( 'NONE',  ( -5.920784292471868326, 6.290491683487167585, 10.00000000000000000 ) ) ;
#7404=CARTESIAN_POINT ( 'NONE',  ( 5.267519402444160725, 2.381954139586888175, 10.00000000000000000 ) ) ;
#7413=CARTESIAN_POINT ( 'NONE',  ( -5.319913005755192437, -3.351504787100450855, 3.747395293195558847E-16 ) ) ;
#7419=CARTESIAN_POINT ( 'NONE',  ( -6.825012239887737309, 1.243808647927286515, 6.857782953271941950E-17 ) ) ;
#7429=CARTESIAN_POINT ( 'NONE',  ( -8.834572391846261752, 1.442725564903824420, 10.00000000000000000 ) ) ;
#7433=CARTESIAN_POINT ( 'NONE',  ( -3.141381368648054284, 10.98006565327106188, 3.747395293195558847E-16 ) ) ;
#7435=CARTESIAN_POINT ( 'NONE',  ( 3.194803811556592876, -2.743189786380903161, 3.747395293195558847E-16 ) ) ;
#7452=CARTESIAN_POINT ( 'NONE',  ( 11.04976219204102783, -11.79656285006036676, 3.747395293195558847E-16 ) ) ;
#7453=CARTESIAN_POINT ( 'NONE',  ( 8.527474615971319949, 0.9793716136081375145, 6.857782953271941950E-17 ) ) ;
#7467=CARTESIAN_POINT ( 'NONE',  ( -7.575117642440518217, -14.74712341115846392, 6.857782953271941950E-17 ) ) ;
#7477=CARTESIAN_POINT ( 'NONE',  ( 6.600721363681033793, -14.58171973507987751, 10.00000000000000000 ) ) ;
#7480=( NAMED_UNIT ( * ) PLANE_ANGLE_UNIT ( ) SI_UNIT ( $, .RADIAN. ) );
#7484=CARTESIAN_POINT ( 'NONE',  ( -15.85416723795449556, 2.087521067385502693, 10.00000000000000000 ) ) ;
#7486=CARTESIAN_POINT ( 'NONE',  ( -4.263796145714473518, -6.152586724582786104, 6.857782953271941950E-17 ) ) ;
#7487=( NAMED_UNIT ( * ) PLANE_ANGLE_UNIT ( ) SI_UNIT ( $, .RADIAN. ) );
#7496=CARTESIAN_POINT ( 'NONE',  ( -8.109405675831295568, 8.372220220303479010, 10.00000000000000000 ) ) ;
#7499=CARTESIAN_POINT ( 'NONE',  ( 9.701579622837702033, -3.641351606116561612, 3.747395293195558847E-16 ) ) ;
#7515=CARTESIAN_POINT ( 'NONE',  ( 2.839002905303027013, -15.63284973865750693, 3.747395293195558847E-16 ) ) ;
#7523=CARTESIAN_POINT ( 'NONE',  ( 4.525508228541173850, -0.2388087992699347017, 10.00000000000000000 ) ) ;
#7529=CARTESIAN_POINT ( 'NONE',  ( 5.312937634500610073, -1.259815497212794400, 10.00000000000000000 ) ) ;
#7538=CARTESIAN_POINT ( 'NONE',  ( -12.61273389267918610, -8.731886703670456384, 10.00000000000000000 ) ) ;
#7542=CARTESIAN_POINT ( 'NONE',  ( -1.999398781552333970, 15.23274265415849626, 10.00000000000000000 ) ) ;
#7554=CARTESIAN_POINT ( 'NONE',  ( -5.773631947676831189, 9.989728373610905265, 10.00000000000000000 ) ) ;
#7555=SHAPE_REPRESENTATION ( 'spring', ( #8474 ), #10565 ) ;
#7556=ADVANCED_FACE ( 'NONE', ( #11124 ), #5620, .F. ) ;
#7559=CARTESIAN_POINT ( 'NONE',  ( -5.359287035703753865, 6.724520318540387009, 3.747395293195558847E-16 ) ) ;
#7560=CARTESIAN_POINT ( 'NONE',  ( 0.5697670706242773386, -3.781298318517893442, 3.747395293195558847E-16 ) ) ;
#7571=CARTESIAN_POINT ( 'NONE',  ( 13.29800827116429573, 3.099979537169514909, 3.747395293195558847E-16 ) ) ;
#7575=CARTESIAN_POINT ( 'NONE',  ( -8.739072045530903665, -14.04184524613901353, 10.00000000000000000 ) ) ;
#7584=CARTESIAN_POINT ( 'NONE',  ( -13.04979933117209256, -0.2127334381860506995, 6.857782953271941950E-17 ) ) ;
#7594=CARTESIAN_POINT ( 'NONE',  ( 3.885483365683945145, 13.62125166200965332, 10.00000000000000000 ) ) ;
#7599=CARTESIAN_POINT ( 'NONE',  ( 9.623984404418655103, 6.889883918979096578, 10.00000000000000000 ) ) ;
#7609=CARTESIAN_POINT ( 'NONE',  ( -5.920784292471868326, 6.290491683487167585, 10.00000000000000000 ) ) ;
#7611=CARTESIAN_POINT ( 'NONE',  ( 1.831757423467612389, 7.960349185506225389, 3.747395293195558847E-16 ) ) ;
#7613=CARTESIAN_POINT ( 'NONE',  ( -7.575117642440518217, -14.74712341115846392, 6.857782953271941950E-17 ) ) ;
#7630=CARTESIAN_POINT ( 'NONE',  ( 0.4634152073531430105, 14.27464310366533340, 3.747395293195558847E-16 ) ) ;
#7637=CARTESIAN_POINT ( 'NONE',  ( 17.50000000000000000, 0.000000000000000000, 10.00000000000000000 ) ) ;
#7649=CARTESIAN_POINT ( 'NONE',  ( 11.14370178440675474, -8.845034901279911210, 6.857782953271941950E-17 ) ) ;
#7653=VECTOR ( 'NONE', #4377, 1000.000000000000000 ) ;
#7660=CARTESIAN_POINT ( 'NONE',  ( 7.795318149608632119, -14.02504990430958998, 10.00000000000000000 ) ) ;
#7664=CARTESIAN_POINT ( 'NONE',  ( 17.24531215409252383, -2.853661713830123237, 6.857782953271941950E-17 ) ) ;
#7668=CARTESIAN_POINT ( 'NONE',  ( 13.06601448280975220, -5.920767845834314258, 10.00000000000000000 ) ) ;
#7679=CARTESIAN_POINT ( 'NONE',  ( -5.541928854458318732, -2.884958602215172974, 10.00000000000000000 ) ) ;
#7682=CARTESIAN_POINT ( 'NONE',  ( 8.329772390959204742, 2.373743296044067641, 10.00000000000000000 ) ) ;
#7685=CARTESIAN_POINT ( 'NONE',  ( -10.47176928358604364, -8.303818807687074255, 6.857782953271941950E-17 ) ) ;
#7698=CARTESIAN_POINT ( 'NONE',  ( -4.046710180314748939, 10.72208681399755292, 3.747395293195558847E-16 ) ) ;
#7701=VERTEX_POINT ( 'NONE', #9595 ) ;
#7704=CARTESIAN_POINT ( 'NONE',  ( -5.683926142426734884, 14.39978054689284193, 10.00000000000000000 ) ) ;
#7715=CARTESIAN_POINT ( 'NONE',  ( -9.080917052262540423, 12.68274194616037320, 6.857782953271941950E-17 ) ) ;
#7722=CARTESIAN_POINT ( 'NONE',  ( -5.318373871714366707, 13.46535835423756566, 10.00000000000000000 ) ) ;
#7727=CARTESIAN_POINT ( 'NONE',  ( 14.54887842078032989, 0.9530482589066729959, 10.00000000000000000 ) ) ;
#7736=CARTESIAN_POINT ( 'NONE',  ( 5.892341078160698409, -4.186101517074010125, 10.00000000000000000 ) ) ;
#7740=CARTESIAN_POINT ( 'NONE',  ( 2.469054641153702434, -10.61194774715159994, 10.00000000000000000 ) ) ;
#7741=CARTESIAN_POINT ( 'NONE',  ( -5.414455899168758357, -12.47541146648942245, 6.857782953271941950E-17 ) ) ;
#7753=CARTESIAN_POINT ( 'NONE',  ( -0.1481022647113159063, -9.773457036294480815, 3.747395293195558847E-16 ) ) ;
#7758=CARTESIAN_POINT ( 'NONE',  ( -1.999398781552333970, 15.23274265415849626, 10.00000000000000000 ) ) ;
#7767=CARTESIAN_POINT ( 'NONE',  ( 12.58137556868280882, 7.823023050434559700, 6.857782953271941950E-17 ) ) ;
#7775=CARTESIAN_POINT ( 'NONE',  ( -9.045553118584756191, -8.482981269325438944, 10.00000000000000000 ) ) ;
#7787=CARTESIAN_POINT ( 'NONE',  ( -1.124919223378054722, -13.71093750358708796, 10.00000000000000000 ) ) ;
#7789=CARTESIAN_POINT ( 'NONE',  ( -13.29946171776798280, 6.562258890817371793, 3.747395293195558847E-16 ) ) ;
#7797=LINE ( 'NONE', #10615, #9681 ) ;
#7798=CARTESIAN_POINT ( 'NONE',  ( -4.763935748647996959, -4.221771024092342728, 10.00000000000000000 ) ) ;
#7800=CARTESIAN_POINT ( 'NONE',  ( 7.334967666341840165, -8.371827447635059372, 10.00000000000000000 ) ) ;
#7803=CARTESIAN_POINT ( 'NONE',  ( -11.80455809908225717, -11.41585333555581627, 6.857782953271941950E-17 ) ) ;
#7807=EDGE_CURVE ( 'NONE', #6584, #4165, #10450, .T. ) ;
#7815=CARTESIAN_POINT ( 'NONE',  ( -7.812220363925484357, -5.053636123081432174, 3.747395293195558847E-16 ) ) ;
#7822=CARTESIAN_POINT ( 'NONE',  ( 8.547432504761534489, 12.33942397201040286, 10.00000000000000000 ) ) ;
#7834=CARTESIAN_POINT ( 'NONE',  ( -11.61414229320030067, -6.453515506896104981, 6.857782953271941950E-17 ) ) ;
#7843=CARTESIAN_POINT ( 'NONE',  ( -0.3758430365714709454, 11.29677535215814466, 10.00000000000000000 ) ) ;
#7851=CARTESIAN_POINT ( 'NONE',  ( -4.389456771235332511, 11.66511648340389762, 10.00000000000000000 ) ) ;
#7853=CARTESIAN_POINT ( 'NONE',  ( -5.318373871714365819, 13.46535835423756389, 3.747395293195558847E-16 ) ) ;
#7856=EDGE_CURVE ( 'NONE', #3870, #1562, #11789, .T. ) ;
#7866=CARTESIAN_POINT ( 'NONE',  ( -10.03906249502029091, -0.8181230654450249995, 10.00000000000000000 ) ) ;
#7868=CARTESIAN_POINT ( 'NONE',  ( -16.00307013876014750, -1.840746716621878498, 6.857782953271941950E-17 ) ) ;
#7880=CARTESIAN_POINT ( 'NONE',  ( 8.429646098664187903, -5.822225404888638600, 3.747395293195558847E-16 ) ) ;
#7886=CARTESIAN_POINT ( 'NONE',  ( -7.327987143158986250, -11.36402271042610224, 10.00000000000000000 ) ) ;
#7895=CARTESIAN_POINT ( 'NONE',  ( 0.6097887191948974106, 9.229167205757265791, 6.857782953271941950E-17 ) ) ;
#7902=CARTESIAN_POINT ( 'NONE',  ( -5.773631947676831189, 9.989728373610905265, 10.00000000000000000 ) ) ;
#7909=CARTESIAN_POINT ( 'NONE',  ( -6.506554845699742629, -8.196137552274390004, 10.00000000000000000 ) ) ;
#7911=CARTESIAN_POINT ( 'NONE',  ( -13.83044629298881034, 5.462350471645222250, 3.747395293195558847E-16 ) ) ;
#7920=CARTESIAN_POINT ( 'NONE',  ( 2.004495162477544223, 5.838205294495796949, 10.00000000000000000 ) ) ;
#7922=CARTESIAN_POINT ( 'NONE',  ( 0.7062845326066684581, -10.79445016380498501, 6.857782953271941950E-17 ) ) ;
#7935=CARTESIAN_POINT ( 'NONE',  ( -9.680665087125342794, -7.686621967951971612, 3.747395293195558847E-16 ) ) ;
#7941=CARTESIAN_POINT ( 'NONE',  ( 12.58137556868281237, 7.823023050435613968, 10.00000000000000000 ) ) ;
#7950=CARTESIAN_POINT ( 'NONE',  ( -9.977213461302312680, -1.645879626164740817, 6.857782953271941950E-17 ) ) ;
#7956=CARTESIAN_POINT ( 'NONE',  ( 9.962304844536470583, 3.945508033568877249, 10.00000000000000000 ) ) ;
#7962=CARTESIAN_POINT ( 'NONE',  ( 5.247589697392150754, -6.187652788349034871, 10.00000000000000000 ) ) ;
#7965=CARTESIAN_POINT ( 'NONE',  ( -11.92955594661033203, -2.174140050202131302, 3.747395293195558847E-16 ) ) ;
#7972=ORIENTED_EDGE ( 'NONE', *, *, #4211, .T. ) ;
#7975=CARTESIAN_POINT ( 'NONE',  ( 3.666996827460253350, 4.772409917195344242, 10.00000000000000000 ) ) ;
#7976=CARTESIAN_POINT ( 'NONE',  ( -0.1504880127286837288, 9.287785325659760005, 6.857782953271941950E-17 ) ) ;
#7983=CARTESIAN_POINT ( 'NONE',  ( 12.25096627321952170, 6.291700371256734314, 10.00000000000000000 ) ) ;
#7987=CARTESIAN_POINT ( 'NONE',  ( 7.527773320476327079, 0.8933511214758176333, 3.747395293195558847E-16 ) ) ;
#7995=CARTESIAN_POINT ( 'NONE',  ( 10.35108484788239203, -9.702746953904565430, 10.00000000000000000 ) ) ;
#8007=CARTESIAN_POINT ( 'NONE',  ( 10.90031251054715966, 4.301772984117409493, 6.857782953271941950E-17 ) ) ;
#8014=CARTESIAN_POINT ( 'NONE',  ( -2.069312577552833154, -12.54440658741724235, 10.00000000000000000 ) ) ;
#8019=PLANE ( 'NONE',  #3768 ) ;
#8021=ORIENTED_EDGE ( 'NONE', *, *, #7807, .T. ) ;
#8024=CARTESIAN_POINT ( 'NONE',  ( -9.352287007200070335, 3.176141031410558924, 10.00000000000000000 ) ) ;
#8028=CARTESIAN_POINT ( 'NONE',  ( 13.03626601087042758, 4.193914020170396384, 3.747395293195558847E-16 ) ) ;
#8044=CARTESIAN_POINT ( 'NONE',  ( -6.266017822847494756, 10.86399168115690728, 6.857782953271941950E-17 ) ) ;
#8045=SURFACE_SIDE_STYLE ('',( #9885 ) ) ;
#8052=CARTESIAN_POINT ( 'NONE',  ( -15.05755265055531389, -0.4891349978715465729, 10.00000000000000000 ) ) ;
#8058=CARTESIAN_POINT ( 'NONE',  ( -6.925491926711623059, 5.292860106065907289, 3.747395293195558847E-16 ) ) ;
#8076=CARTESIAN_POINT ( 'NONE',  ( -2.764021070441483374, -10.29567250283335689, 6.857782953271941950E-17 ) ) ;
#8083=CARTESIAN_POINT ( 'NONE',  ( 7.261170810407329590, -1.543028577657542311, 10.00000000000000000 ) ) ;
#8086=CARTESIAN_POINT ( 'NONE',  ( 0.0002901587068754535662, -4.749354241797641762, 5.000000000000000000 ) ) ;
#8092=CARTESIAN_POINT ( 'NONE',  ( -9.820986981723351050, 1.626514086989862662, 10.00000000000000000 ) ) ;
#8095=CARTESIAN_POINT ( 'NONE',  ( 12.25096627321951814, 6.291700371256212065, 3.747395293195558847E-16 ) ) ;
#8100=CARTESIAN_POINT ( 'NONE',  ( -6.036922680726758195, -0.4347383792561972382, 3.747395293195558847E-16 ) ) ;
#8108=CARTESIAN_POINT ( 'NONE',  ( 5.531377455021724288, -0.3672033614207039776, 10.00000000000000000 ) ) ;
#8109=CARTESIAN_POINT ( 'NONE',  ( -4.368568794346921358, -9.638580752213396607, 6.857782953271941950E-17 ) ) ;
#8116=CARTESIAN_POINT ( 'NONE',  ( -13.25288834650809910, -7.646628085889272342, 10.00000000000000000 ) ) ;
#8121=CARTESIAN_POINT ( 'NONE',  ( -3.432991321284826647, 4.402131891631369420, 3.747395293195558847E-16 ) ) ;
#8136=CARTESIAN_POINT ( 'NONE',  ( -4.859750766526011567, 4.557676925202717833, 6.857782953271941950E-17 ) ) ;
#8143=CARTESIAN_POINT ( 'NONE',  ( -8.834572391846261752, 1.442725564903824420, 10.00000000000000000 ) ) ;
#8149=CARTESIAN_POINT ( 'NONE',  ( 2.919619825260427071, -7.400844473264730716, 10.00000000000000000 ) ) ;
#8158=CARTESIAN_POINT ( 'NONE',  ( -5.315861670734002509, 2.363279591655833567, 3.747395293195558847E-16 ) ) ;
#8164=CARTESIAN_POINT ( 'NONE',  ( 4.346347989804005607, 4.041826679702273495, 10.00000000000000000 ) ) ;
#8165=CARTESIAN_POINT ( 'NONE',  ( -3.406233159845096559, 11.94786423299364486, 6.857782953271941950E-17 ) ) ;
#8172=CARTESIAN_POINT ( 'NONE',  ( 3.885483365683945145, 13.62125166200965332, 10.00000000000000000 ) ) ;
#8178=CARTESIAN_POINT ( 'NONE',  ( 7.402789038520869447, -0.9464297003978341394, 3.747395293195558847E-16 ) ) ;
#8195=CARTESIAN_POINT ( 'NONE',  ( -0.5113267480521395125, 6.289062763288773894, 6.857782953271941950E-17 ) ) ;
#8202=CARTESIAN_POINT ( 'NONE',  ( 0.9209971296404340091, -6.773236541304583191, 10.00000000000000000 ) ) ;
#8210=CARTESIAN_POINT ( 'NONE',  ( 0.6279411196271856843, -4.781877258324073843, 10.00000000000000000 ) ) ;
#8216=CARTESIAN_POINT ( 'NONE',  ( 5.657123057053811799, 5.504982807385217392, 3.747395293195558847E-16 ) ) ;
#8226=CARTESIAN_POINT ( 'NONE',  ( -8.739072045530903665, -14.04184524613901353, 10.00000000000000000 ) ) ;
#8227=CARTESIAN_POINT ( 'NONE',  ( 4.764169229608189227, 7.652272242164855243, 6.857782953271941950E-17 ) ) ;
#8238=CARTESIAN_POINT ( 'NONE',  ( 12.96212312671954514, -3.473279994529783199, 10.00000000000000000 ) ) ;
#8243=CARTESIAN_POINT ( 'NONE',  ( -3.663109177303993214, -5.348850660921103284, 3.747395293195558847E-16 ) ) ;
#8258=CARTESIAN_POINT ( 'NONE',  ( 8.235329212250112718, -1.783486464602660027, 6.857782953271941950E-17 ) ) ;
#8267=CARTESIAN_POINT ( 'NONE',  ( 1.482756436301465808, -6.713508106970953015, 10.00000000000000000 ) ) ;
#8277=CARTESIAN_POINT ( 'NONE',  ( -14.12277927129995803, -8.146689865454474599, 6.857782953271941950E-17 ) ) ;
#8284=CARTESIAN_POINT ( 'NONE',  ( 5.892341078160108658, -4.186101517074008349, 3.747395293195558847E-16 ) ) ;
#8291=CARTESIAN_POINT ( 'NONE',  ( 7.252227276001472767, 5.017415995114415495, 6.857782953271941950E-17 ) ) ;
#8299=CARTESIAN_POINT ( 'NONE',  ( 2.257301671556971367, -9.631158585656901749, 10.00000000000000000 ) ) ;
#8303=CARTESIAN_POINT ( 'NONE',  ( 4.889075487039526990, 9.929493272050624597, 3.747395293195558847E-16 ) ) ;
#8306=CARTESIAN_POINT ( 'NONE',  ( 0.8073695008816142993, 5.181225205791315958, 3.747395293195558847E-16 ) ) ;
#8321=CARTESIAN_POINT ( 'NONE',  ( -14.85975435031504510, 1.953672781916663936, 3.747395293195558847E-16 ) ) ;
#8322=CARTESIAN_POINT ( 'NONE',  ( 2.919619825260425294, -7.400844473264723611, 6.857782953271941950E-17 ) ) ;
#8330=CARTESIAN_POINT ( 'NONE',  ( -3.038216613430223756, 4.635879136410493651, 10.00000000000000000 ) ) ;
#8337=CARTESIAN_POINT ( 'NONE',  ( -6.191802569540381995, -3.848120238388911041, 10.00000000000000000 ) ) ;
#8346=CARTESIAN_POINT ( 'NONE',  ( 1.482756436301464920, -6.713508106970949463, 3.747395293195558847E-16 ) ) ;
#8354=CARTESIAN_POINT ( 'NONE',  ( 0.0002901587068756704066, -4.749354241797638210, 6.857782953271941950E-17 ) ) ;
#8355=( NAMED_UNIT ( * ) SI_UNIT ( $, .STERADIAN. ) SOLID_ANGLE_UNIT ( ) );
#8360=CARTESIAN_POINT ( 'NONE',  ( 1.454091968623351550, 11.13059540125182778, 10.00000000000000000 ) ) ;
#8363=CARTESIAN_POINT ( 'NONE',  ( -9.037587479195730467, -0.7561632655184011842, 3.747395293195558847E-16 ) ) ;
#8381=CARTESIAN_POINT ( 'NONE',  ( 9.623054350189519823, -9.012277985855606133, 3.747395293195558847E-16 ) ) ;
#8382=CARTESIAN_POINT ( 'NONE',  ( -4.263796145714473518, -6.152586724582786104, 6.857782953271941950E-17 ) ) ;
#8397=CARTESIAN_POINT ( 'NONE',  ( -8.739072045530900112, -14.04184524613900820, 6.857782953271941950E-17 ) ) ;
#8406=CARTESIAN_POINT ( 'NONE',  ( -11.99326810842507562, 8.590522060507204571, 10.00000000000000000 ) ) ;
#8412=CARTESIAN_POINT ( 'NONE',  ( -7.575117642440520882, -14.74712341115847103, 10.00000000000000000 ) ) ;
#8414=CARTESIAN_POINT ( 'NONE',  ( 5.247589697392725405, -6.187652788349031319, 6.857782953271941950E-17 ) ) ;
#8426=CARTESIAN_POINT ( 'NONE',  ( -8.409270314015810044, 2.833341551407463133, 10.00000000000000000 ) ) ;
#8431=CARTESIAN_POINT ( 'NONE',  ( -4.046710180314748939, 10.72208681399755292, 3.747395293195558847E-16 ) ) ;
#8449=CARTESIAN_POINT ( 'NONE',  ( 7.081399987883180813, -10.98142027556026612, 3.747395293195558847E-16 ) ) ;
#8467=CARTESIAN_POINT ( 'NONE',  ( 7.014224211608840243, -15.49593329755746218, 6.857782953271941950E-17 ) ) ;
#8468=DIRECTION ( 'NONE',  ( -0.07332096784668425127, -0.9973083954695386444, 0.000000000000000000 ) ) ;
#8474=AXIS2_PLACEMENT_3D ( 'NONE', #1674, #1551, #2653 ) ;
#8475=CARTESIAN_POINT ( 'NONE',  ( -14.85975435031504865, 1.953672781916663936, 10.00000000000000000 ) ) ;
#8481=CARTESIAN_POINT ( 'NONE',  ( -15.56595607421884075, -4.438723023272252988, 10.00000000000000000 ) ) ;
#8483=CARTESIAN_POINT ( 'NONE',  ( -5.152979166089614260, -5.321787192520350374, 6.857782953271941950E-17 ) ) ;
#8491=CARTESIAN_POINT ( 'NONE',  ( 4.583115687978493114, -8.898851689027766909, 10.00000000000000000 ) ) ;
#8492=DIRECTION ( 'NONE',  ( 1.000000000000000000, -0.000000000000000000, -0.000000000000000000 ) ) ;
#8493=CARTESIAN_POINT ( 'NONE',  ( -1.515734900794040385, 8.225284064336934264, 3.747395293195558847E-16 ) ) ;
#8509=CARTESIAN_POINT ( 'NONE',  ( 4.163410377374355598, -12.26152398776834040, 3.747395293195558847E-16 ) ) ;
#8513=CARTESIAN_POINT ( 'NONE',  ( -15.59049818040342927, 3.373450308083567606, 10.00000000000000000 ) ) ;
#8521=CARTESIAN_POINT ( 'NONE',  ( -12.72059027619867244, -3.407653011835690471, 6.857782953271941950E-17 ) ) ;
#8529=CARTESIAN_POINT ( 'NONE',  ( 15.52845182490561626, -5.270724383582042982, 10.00000000000000000 ) ) ;
#8534=CARTESIAN_POINT ( 'NONE',  ( 13.92981926110968161, -3.738495919395732781, 10.00000000000000000 ) ) ;
#8547=CARTESIAN_POINT ( 'NONE',  ( -7.812220363924760491, -5.053636123081433951, 10.00000000000000000 ) ) ;
#8549=CARTESIAN_POINT ( 'NONE',  ( -2.196651480121880162, 8.111327970581170277, 3.747395293195558847E-16 ) ) ;
#8550=CARTESIAN_POINT ( 'NONE',  ( 13.14573027368987646, 6.745762002080606834, 6.857782953271941950E-17 ) ) ;
#8553=ORIENTED_EDGE ( 'NONE', *, *, #4533, .F. ) ;
#8563=CARTESIAN_POINT ( 'NONE',  ( 3.885483365683944257, 13.62125166200964976, 3.747395293195558847E-16 ) ) ;
#8569=CARTESIAN_POINT ( 'NONE',  ( 16.47843063274657993, -5.593696103119286001, 10.00000000000000000 ) ) ;
#8578=CARTESIAN_POINT ( 'NONE',  ( -6.266017822847494756, 10.86399168115690728, 6.857782953271941950E-17 ) ) ;
#8588=CARTESIAN_POINT ( 'NONE',  ( -13.25288834650809910, -7.646628085889272342, 10.00000000000000000 ) ) ;
#8591=CARTESIAN_POINT ( 'NONE',  ( 13.67726327739689829, -10.50289975150003485, 6.857782953271941950E-17 ) ) ;
#8594=CARTESIAN_POINT ( 'NONE',  ( 2.578468386369561216, 11.91291369680097567, 10.00000000000000000 ) ) ;
#8605=CARTESIAN_POINT ( 'NONE',  ( 3.120778274233608318, -6.257845451232916467, 10.00000000000000000 ) ) ;
#8610=CARTESIAN_POINT ( 'NONE',  ( 5.027256439335601179, -9.798587832406491671, 10.00000000000000000 ) ) ;
#8611=CARTESIAN_POINT ( 'NONE',  ( -15.56595607421883365, -4.438723023272252100, 6.857782953271941950E-17 ) ) ;
#8625=CARTESIAN_POINT ( 'NONE',  ( -11.92955594661033203, -2.174140050202131302, 3.747395293195558847E-16 ) ) ;
#8630=CARTESIAN_POINT ( 'NONE',  ( -14.12277927129996158, -8.146689865454478152, 10.00000000000000000 ) ) ;
#8641=CARTESIAN_POINT ( 'NONE',  ( 8.588976300537435549, -11.19439025337200810, 6.857782953271941950E-17 ) ) ;
#8651=CARTESIAN_POINT ( 'NONE',  ( -8.207979594962568015, -13.19054478262514607, 10.00000000000000000 ) ) ;
#8660=CARTESIAN_POINT ( 'NONE',  ( 11.50231346626665996, 1.508968394323198847, 10.00000000000000000 ) ) ;
#8662=CARTESIAN_POINT ( 'NONE',  ( -15.05755265055531034, -0.4891349978715467950, 3.747395293195558847E-16 ) ) ;
#8669=CARTESIAN_POINT ( 'NONE',  ( -0.1881845630465191765, -6.755137126427050553, 10.00000000000000000 ) ) ;
#8672=CARTESIAN_POINT ( 'NONE',  ( 7.449730884303676248, -3.679036338562946096, 10.00000000000000000 ) ) ;
#8673=CARTESIAN_POINT ( 'NONE',  ( 11.14370178440675474, -8.845034901279911210, 6.857782953271941950E-17 ) ) ;
#8687=CARTESIAN_POINT ( 'NONE',  ( -11.32214898804403802, 3.633524203738173419, 3.747395293195558847E-16 ) ) ;
#8695=CARTESIAN_POINT ( 'NONE',  ( -6.864300873105356082, 13.92024697337932082, 10.00000000000000000 ) ) ;
#8698=CARTESIAN_POINT ( 'NONE',  ( 11.73504485001147124, -12.52947377801878837, 6.857782953271941950E-17 ) ) ;
#8705=CARTESIAN_POINT ( 'NONE',  ( -4.384918567263694555, -12.91535881965570631, 6.857782953271941950E-17 ) ) ;
#8711=CARTESIAN_POINT ( 'NONE',  ( -1.307086582043127443, 11.26718560147321568, 10.00000000000000000 ) ) ;
#8716=CARTESIAN_POINT ( 'NONE',  ( -12.27443204882852257, 3.949650873796767492, 10.00000000000000000 ) ) ;
#8719=CARTESIAN_POINT ( 'NONE',  ( -15.00596061316373842, -1.728743269517114323, 3.747395293195558847E-16 ) ) ;
#8727=CARTESIAN_POINT ( 'NONE',  ( 0.9209971296404340091, -6.773236541304583191, 10.00000000000000000 ) ) ;
#8731=CARTESIAN_POINT ( 'NONE',  ( -9.023584016175229650, 3.917288190900558131, 10.00000000000000000 ) ) ;
#8732=CARTESIAN_POINT ( 'NONE',  ( -13.04979933117209256, -0.2127334381860506995, 6.857782953271941950E-17 ) ) ;
#8742=CARTESIAN_POINT ( 'NONE',  ( -4.622662292628548997, -8.344572748942098883, 3.747395293195558847E-16 ) ) ;
#8759=CARTESIAN_POINT ( 'NONE',  ( -1.999398781552333526, 15.23274265415848916, 6.857782953271941950E-17 ) ) ;
#8765=CARTESIAN_POINT ( 'NONE',  ( -2.487495860704070250, -9.331140650584721641, 10.00000000000000000 ) ) ;
#8769=VECTOR ( 'NONE', #10009, 1000.000000000000227 ) ;
#8773=CARTESIAN_POINT ( 'NONE',  ( -9.546882484473293573, 8.373557015401750903, 10.00000000000000000 ) ) ;
#8774=CARTESIAN_POINT ( 'NONE',  ( -4.793139000956299967, -14.90149022103882892, 3.747395293195558847E-16 ) ) ;
#8785=CARTESIAN_POINT ( 'NONE',  ( -2.764021070441486039, -10.29567250283336399, 10.00000000000000000 ) ) ;
#8788=CARTESIAN_POINT ( 'NONE',  ( 13.92981926110967450, -3.738495919395730116, 6.857782953271941950E-17 ) ) ;
#8796=CARTESIAN_POINT ( 'NONE',  ( 16.25531780653859570, -2.690316503436296802, 10.00000000000000000 ) ) ;
#8800=CARTESIAN_POINT ( 'NONE',  ( -8.109405675832187299, 8.372220220304370741, 3.747395293195558847E-16 ) ) ;
#8807=CARTESIAN_POINT ( 'NONE',  ( -3.406233159845097891, 11.94786423299365197, 10.00000000000000000 ) ) ;
#8815=EDGE_LOOP ( 'NONE', ( #8553, #7972, #11634, #5870 ) ) ;
#8819=CARTESIAN_POINT ( 'NONE',  ( -9.820986981721938847, 1.626514086989861108, 6.857782953271941950E-17 ) ) ;
#8827=CARTESIAN_POINT ( 'NONE',  ( -8.694522232909452697, -2.966707450564700643, 10.00000000000000000 ) ) ;
#8836=CARTESIAN_POINT ( 'NONE',  ( 8.143984375790578767, 3.063465613658708619, 10.00000000000000000 ) ) ;
#8850=CARTESIAN_POINT ( 'NONE',  ( 2.798030692817974341, 8.692477993603725750, 10.00000000000000000 ) ) ;
#8852=CARTESIAN_POINT ( 'NONE',  ( 11.51680056346191883, -0.3781118375584790470, 6.857782953271941950E-17 ) ) ;
#8863=CARTESIAN_POINT ( 'NONE',  ( 10.00611923916670953, -2.842981073525689517, 3.747395293195558847E-16 ) ) ;
#8871=CARTESIAN_POINT ( 'NONE',  ( -1.124919223378054722, -13.71093750358708796, 10.00000000000000000 ) ) ;
#8881=CARTESIAN_POINT ( 'NONE',  ( 8.329772390959197637, 2.373743296044066309, 6.857782953271941950E-17 ) ) ;
#8887=CARTESIAN_POINT ( 'NONE',  ( -6.777230418910823673, -10.52530689671158548, 10.00000000000000000 ) ) ;
#8893=CARTESIAN_POINT ( 'NONE',  ( 8.527474615971327054, 0.9793716136081388468, 10.00000000000000000 ) ) ;
#8895=CARTESIAN_POINT ( 'NONE',  ( -11.15100792855598755, -5.055838994807843711, 3.747395293195558847E-16 ) ) ;
#8901=LINE ( 'NONE', #2345, #2650 ) ;
#8907=CARTESIAN_POINT ( 'NONE',  ( 5.247589697392150754, -6.187652788349034871, 10.00000000000000000 ) ) ;
#8908=CARTESIAN_POINT ( 'NONE',  ( -5.965338750500049692, 7.524205049158500636, 6.857782953271941950E-17 ) ) ;
#8916=CARTESIAN_POINT ( 'NONE',  ( -4.793139000956300855, -14.90149022103883247, 10.00000000000000000 ) ) ;
#8920=CARTESIAN_POINT ( 'NONE',  ( 0.9209971296404340091, -6.773236541304579639, 3.747395293195558847E-16 ) ) ;
#8926=CARTESIAN_POINT ( 'NONE',  ( 11.14370178440676007, -8.845034901279914763, 10.00000000000000000 ) ) ;
#8937=CARTESIAN_POINT ( 'NONE',  ( -9.386162357322611172, -4.067606288967436257, 6.857782953271941950E-17 ) ) ;
#8942=CARTESIAN_POINT ( 'NONE',  ( -11.74902089294173813, -3.156991809147611683, 10.00000000000000000 ) ) ;
#8947=CARTESIAN_POINT ( 'NONE',  ( 1.661435237661583297, -7.700870200009183542, 10.00000000000000000 ) ) ;
#8951=CARTESIAN_POINT ( 'NONE',  ( -10.51222845931327576, 5.388985543800765221, 3.747395293195558847E-16 ) ) ;
#8962=CARTESIAN_POINT ( 'NONE',  ( 2.084091085258986009, 8.931495281877380066, 6.857782953271941950E-17 ) ) ;
#8971=CARTESIAN_POINT ( 'NONE',  ( 9.623054350189521600, -9.012277985855607909, 10.00000000000000000 ) ) ;
#8975=CARTESIAN_POINT ( 'NONE',  ( -8.962830026514755133, 0.7152994853347065529, 3.747395293195558847E-16 ) ) ;
#8982=CARTESIAN_POINT ( 'NONE',  ( 2.259453438922059298, -13.68937604509904737, 10.00000000000000000 ) ) ;
#8986=CARTESIAN_POINT ( 'NONE',  ( 1.445324715877977173, -3.701599742324200637, 10.00000000000000000 ) ) ;
#8994=CARTESIAN_POINT ( 'NONE',  ( 5.343773788080180331, 10.82393792025543711, 6.857782953271941950E-17 ) ) ;
#9001=CARTESIAN_POINT ( 'NONE',  ( 2.581500635392915299, -6.456130005640037695, 10.00000000000000000 ) ) ;
#9009=CARTESIAN_POINT ( 'NONE',  ( -0.1814876354083667931, -10.77628937513455654, 10.00000000000000000 ) ) ;
#9012=CARTESIAN_POINT ( 'NONE',  ( 1.050035089571674352, -12.78847817906846096, 3.747395293195558847E-16 ) ) ;
#9025=EDGE_CURVE ( 'NONE', #7701, #5043, #4932, .T. ) ;
#9030=CARTESIAN_POINT ( 'NONE',  ( -6.589974825828272209, 7.038139701356662670, 6.857782953271941950E-17 ) ) ;
#9037=CARTESIAN_POINT ( 'NONE',  ( -11.92955594661033558, -2.174140050202246766, 10.00000000000000000 ) ) ;
#9042=CARTESIAN_POINT ( 'NONE',  ( -5.069009347565034851, 2.772702716244574095, 3.747395293195558847E-16 ) ) ;
#9059=CARTESIAN_POINT ( 'NONE',  ( 1.597090680284417363, 12.12373805211590749, 6.857782953271941950E-17 ) ) ;
#9069=CARTESIAN_POINT ( 'NONE',  ( -5.846204292276370396, 1.022993486932170404, 10.00000000000000000 ) ) ;
#9074=CARTESIAN_POINT ( 'NONE',  ( 4.698850784960275639, -6.565226861933597391, 10.00000000000000000 ) ) ;
#9083=CARTESIAN_POINT ( 'NONE',  ( -4.428608208598374674, -4.627450663480007442, 3.747395293195558847E-16 ) ) ;
#9089=CARTESIAN_POINT ( 'NONE',  ( 1.018538006779725835, -7.771884277300785904, 10.00000000000000000 ) ) ;
#9090=CARTESIAN_POINT ( 'NONE',  ( -6.506554845699739076, -8.196137552275128968, 6.857782953271941950E-17 ) ) ;
#9096=CARTESIAN_POINT ( 'NONE',  ( 7.081399987883182590, -10.98142027556026967, 10.00000000000000000 ) ) ;
#9100=CARTESIAN_POINT ( 'NONE',  ( -5.315861670734002509, 2.363279591655833567, 3.747395293195558847E-16 ) ) ;
#9108=CARTESIAN_POINT ( 'NONE',  ( 3.194803811556594653, -2.743189786380181072, 10.00000000000000000 ) ) ;
#9114=CARTESIAN_POINT ( 'NONE',  ( -7.014275365397503847, 0.1192422097806469378, 6.857782953271941950E-17 ) ) ;
#9120=CARTESIAN_POINT ( 'NONE',  ( -8.409270314015810044, 2.833341551407463133, 10.00000000000000000 ) ) ;
#9128=CARTESIAN_POINT ( 'NONE',  ( -7.040021908109685533, -0.4595208068205508534, 10.00000000000000000 ) ) ;
#9135=CARTESIAN_POINT ( 'NONE',  ( 5.211919109253432936, 5.981019939437269173, 3.747395293195558847E-16 ) ) ;
#9140=CARTESIAN_POINT ( 'NONE',  ( -0.2556890074706391625, -7.756263830888999067, 10.00000000000000000 ) ) ;
#9142=CARTESIAN_POINT ( 'NONE',  ( -6.947552178111042309, -1.615339808524891563, 6.857782953271941950E-17 ) ) ;
#9149=CARTESIAN_POINT ( 'NONE',  ( 7.972781652389874907, 11.51689705412746711, 10.00000000000000000 ) ) ;
#9153=CARTESIAN_POINT ( 'NONE',  ( -5.920784292472551336, 6.290491683487165808, 3.747395293195558847E-16 ) ) ;
#9175=CARTESIAN_POINT ( 'NONE',  ( -4.158289900078591117, 7.437556212722741478, 10.00000000000000000 ) ) ;
#9181=CARTESIAN_POINT ( 'NONE',  ( 11.73504485001147124, -12.52947377801878837, 6.857782953271941950E-17 ) ) ;
#9190=CARTESIAN_POINT ( 'NONE',  ( -0.9167995209625431352, 5.268308710424121521, 3.747395293195558847E-16 ) ) ;
#9200=CARTESIAN_POINT ( 'NONE',  ( 17.46093749967478814, -1.431715403549062904, 10.00000000000000000 ) ) ;
#9203=CARTESIAN_POINT ( 'NONE',  ( -0.5113267480521395125, 6.289062763288773894, 6.857782953271941950E-17 ) ) ;
#9204=PRODUCT_DEFINITION_FORMATION_WITH_SPECIFIED_SOURCE ( 'ANY', '', #18, .NOT_KNOWN. ) ;
#9205=( LENGTH_UNIT ( ) NAMED_UNIT ( * ) SI_UNIT ( .MILLI., .METRE. ) );
#9215=CARTESIAN_POINT ( 'NONE',  ( -6.597323627732286866, 9.514359934152452070, 10.00000000000000000 ) ) ;
#9220=CARTESIAN_POINT ( 'NONE',  ( 9.640149279600553456, 4.768118462334743235, 3.747395293195558847E-16 ) ) ;
#9233=DIRECTION ( 'NONE',  ( -1.000000000000000000, 0.000000000000000000, 3.061616997868383141E-16 ) ) ;
#9236=CARTESIAN_POINT ( 'NONE',  ( -7.115032382426029756, -13.85544350050026452, 3.747395293195558847E-16 ) ) ;
#9245=CARTESIAN_POINT ( 'NONE',  ( -5.069009347565514467, 2.772702716245054155, 10.00000000000000000 ) ) ;
#9253=CARTESIAN_POINT ( 'NONE',  ( -5.152979166089619589, -5.321787192520355703, 10.00000000000000000 ) ) ;
#9260=CARTESIAN_POINT ( 'NONE',  ( 6.841929108544086091, -2.672872603904024480, 3.747395293195558847E-16 ) ) ;
#9266=CARTESIAN_POINT ( 'NONE',  ( 17.50000000000000000, 0.000000000000000000, 10.00000000000000000 ) ) ;
#9267=CARTESIAN_POINT ( 'NONE',  ( 1.737537816361722331, -4.672682311025833535, 6.857782953271941950E-17 ) ) ;
#9275=PRODUCT_DEFINITION ( 'UNKNOWN', '', #9204, #3294 ) ;
#9277=CARTESIAN_POINT ( 'NONE',  ( 0.5199114366211746718, 8.229807867079658834, 10.00000000000000000 ) ) ;
#9282=CARTESIAN_POINT ( 'NONE',  ( 10.39479819782869541, 2.258419626871296604, 3.747395293195558847E-16 ) ) ;
#9296=CARTESIAN_POINT ( 'NONE',  ( 12.96212312671852551, -3.473279994529273829, 3.747395293195558847E-16 ) ) ;
#9297=CARTESIAN_POINT ( 'NONE',  ( 1.661435237661581521, -7.700870200009177324, 6.857782953271941950E-17 ) ) ;
#9313=CARTESIAN_POINT ( 'NONE',  ( -5.101271054653079950, -15.85638610327790765, 6.857782953271941950E-17 ) ) ;
#9321=CARTESIAN_POINT ( 'NONE',  ( 1.631735293711819246, 4.895207720155139164, 3.747395293195558847E-16 ) ) ;
#9327=CARTESIAN_POINT ( 'NONE',  ( -6.191802569540376666, -3.848120238389427072, 6.857782953271941950E-17 ) ) ;
#9335=CARTESIAN_POINT ( 'NONE',  ( 7.078846155420733588, 8.354583459611244933, 10.00000000000000000 ) ) ;
#9339=CARTESIAN_POINT ( 'NONE',  ( -8.984113827416486231, -1.502549133976348372, 3.747395293195558847E-16 ) ) ;
#9353=CARTESIAN_POINT ( 'NONE',  ( 10.44364468045615801, 9.157203537817473205, 3.747395293195558847E-16 ) ) ;
#9354=CARTESIAN_POINT ( 'NONE',  ( 3.913389251770639010, -3.458713887698550593, 6.857782953271941950E-17 ) ) ;
#9371=CARTESIAN_POINT ( 'NONE',  ( 1.737537816361723220, -4.672682311025840640, 10.00000000000000000 ) ) ;
#9378=CARTESIAN_POINT ( 'NONE',  ( 7.972781652389874907, 11.51689705412746711, 10.00000000000000000 ) ) ;
#9386=CARTESIAN_POINT ( 'NONE',  ( -0.8869411547437818788, -7.669649013129171244, 6.857782953271941950E-17 ) ) ;
#9395=CARTESIAN_POINT ( 'NONE',  ( -2.487495860704070250, -9.331140650584721641, 10.00000000000000000 ) ) ;
#9399=CARTESIAN_POINT ( 'NONE',  ( 5.319643049700911952, -8.526005966358411570, 3.747395293195558847E-16 ) ) ;
#9416=CARTESIAN_POINT ( 'NONE',  ( -4.793139000956299967, -14.90149022103882892, 3.747395293195558847E-16 ) ) ;
#9424=CARTESIAN_POINT ( 'NONE',  ( 14.52660474336370200, -9.366294961249359119, 10.00000000000000000 ) ) ;
#9434=CARTESIAN_POINT ( 'NONE',  ( -16.00307013876014750, -1.840746716621878498, 6.857782953271941950E-17 ) ) ;
#9442=CARTESIAN_POINT ( 'NONE',  ( 16.25531780653859570, -2.690316503436296802, 10.00000000000000000 ) ) ;
#9448=CARTESIAN_POINT ( 'NONE',  ( -14.76245309360257174, 5.834016798581408203, 10.00000000000000000 ) ) ;
#9451=CARTESIAN_POINT ( 'NONE',  ( -3.791520748785365491, -16.26028641251512497, 6.857782953271941950E-17 ) ) ;
#9460=CARTESIAN_POINT ( 'NONE',  ( 6.391761267591818729, 8.940137919804724831, 10.00000000000000000 ) ) ;
#9462=CARTESIAN_POINT ( 'NONE',  ( -6.430932688512553064, -6.885836206077581068, 3.747395293195558847E-16 ) ) ;
#9463=CARTESIAN_POINT ( 'NONE',  ( -12.27443204883033623, 3.949650873796764827, 6.857782953271941950E-17 ) ) ;
#9477=CARTESIAN_POINT ( 'NONE',  ( 16.25531780653859215, -2.690316503436295914, 3.747395293195558847E-16 ) ) ;
#9482=CARTESIAN_POINT ( 'NONE',  ( -16.06046882360140060, -0.5196555361422392494, 10.00000000000000000 ) ) ;
#9490=CARTESIAN_POINT ( 'NONE',  ( -7.327987143158983585, -11.36402271042705614, 6.857782953271941950E-17 ) ) ;
#9500=CARTESIAN_POINT ( 'NONE',  ( -11.08238827499401680, -10.71925978067563001, 10.00000000000000000 ) ) ;
#9504=CARTESIAN_POINT ( 'NONE',  ( -8.799721882313775723, 9.100398320382247164, 10.00000000000000000 ) ) ;
#9507=CARTESIAN_POINT ( 'NONE',  ( -14.60057116351879714, -4.165219547604622541, 3.747395293195558847E-16 ) ) ;
#9516=CARTESIAN_POINT ( 'NONE',  ( 4.140589500486091090, -5.731468560951012314, 10.00000000000000000 ) ) ;
#9519=CARTESIAN_POINT ( 'NONE',  ( 4.138106518799270717, 8.052838533163344081, 10.00000000000000000 ) ) ;
#9520=CARTESIAN_POINT ( 'NONE',  ( 12.50121531544688480, -6.953993600215016002, 6.857782953271941950E-17 ) ) ;
#9535=CARTESIAN_POINT ( 'NONE',  ( -7.594692469639082510, -9.901549393537251831, 3.747395293195558847E-16 ) ) ;
#9541=CARTESIAN_POINT ( 'NONE',  ( -16.00307013876015461, -1.840746716621879830, 10.00000000000000000 ) ) ;
#9547=CARTESIAN_POINT ( 'NONE',  ( 17.49999999999999645, 0.000000000000000000, 5.000000000000000000 ) ) ;
#9551=CARTESIAN_POINT ( 'NONE',  ( -4.389456771235329846, 11.66511648340389051, 6.857782953271941950E-17 ) ) ;
#9561=CARTESIAN_POINT ( 'NONE',  ( 13.29800827116429929, 3.099979537169774257, 10.00000000000000000 ) ) ;
#9566=CARTESIAN_POINT ( 'NONE',  ( 10.54603994011899459, 5.199563424939650957, 10.00000000000000000 ) ) ;
#9568=CARTESIAN_POINT ( 'NONE',  ( 13.68367311611256554, -8.822018488634762790, 3.747395293195558847E-16 ) ) ;
#9578=CARTESIAN_POINT ( 'NONE',  ( -5.069009347565514467, 2.772702716245054155, 10.00000000000000000 ) ) ;
#9583=CARTESIAN_POINT ( 'NONE',  ( 9.056240860197965148, 7.682302481599247557, 10.00000000000000000 ) ) ;
#9584=CARTESIAN_POINT ( 'NONE',  ( -1.999398781552333526, 15.23274265415848916, 6.857782953271941950E-17 ) ) ;
#9595=CARTESIAN_POINT ( 'NONE',  ( 16.50000000000000355, 0.000000000000000000, 10.00000000000000000 ) ) ;
#9597=CARTESIAN_POINT ( 'NONE',  ( 6.391761267590965190, 8.940137919805573929, 3.747395293195558847E-16 ) ) ;
#9602=CARTESIAN_POINT ( 'NONE',  ( 7.014224211608842907, -15.49593329755746929, 10.00000000000000000 ) ) ;
#9614=CARTESIAN_POINT ( 'NONE',  ( -15.59049818040117152, 3.373450308083002724, 6.857782953271941950E-17 ) ) ;
#9623=CARTESIAN_POINT ( 'NONE',  ( 1.050035089571674352, -12.78847817906846451, 10.00000000000000000 ) ) ;
#9628=CARTESIAN_POINT ( 'NONE',  ( 10.38524206949726469, 10.73010674553377797, 10.00000000000000000 ) ) ;
#9638=CARTESIAN_POINT ( 'NONE',  ( 5.211919109253434712, 5.981019939437272726, 10.00000000000000000 ) ) ;
#9641=CARTESIAN_POINT ( 'NONE',  ( 8.025946968469186871, -7.769110617520879281, 10.00000000000000000 ) ) ;
#9643=CARTESIAN_POINT ( 'NONE',  ( -11.98007164540816838, 10.17225797950327681, 6.857782953271941950E-17 ) ) ;
#9651=CARTESIAN_POINT ( 'NONE',  ( 16.50000000000000355, 0.000000000000000000, 10.00000000000000000 ) ) ;
#9653=CARTESIAN_POINT ( 'NONE',  ( -1.103316172498963521, -16.73802372459124044, 6.857782953271941950E-17 ) ) ;
#9657=CARTESIAN_POINT ( 'NONE',  ( -1.719633853164446613, -9.543036404944416518, 3.747395293195558847E-16 ) ) ;
#9661=ORIENTED_EDGE ( 'NONE', *, *, #213, .T. ) ;
#9662=CARTESIAN_POINT ( 'NONE',  ( 10.64229886435067840, -13.41933351754447834, 10.00000000000000000 ) ) ;
#9673=CARTESIAN_POINT ( 'NONE',  ( -12.98359546555289334, 0.8565524458115012507, 6.857782953271941950E-17 ) ) ;
#9679=CARTESIAN_POINT ( 'NONE',  ( 4.583115687978493114, -8.898851689027766909, 10.00000000000000000 ) ) ;
#9681=VECTOR ( 'NONE', #7045, 1000.000000000000000 ) ;
#9682=FILL_AREA_STYLE_COLOUR ( '', #11731 ) ;
#9686=CARTESIAN_POINT ( 'NONE',  ( -7.327987143158986250, -11.36402271042610224, 10.00000000000000000 ) ) ;
#9688=CARTESIAN_POINT ( 'NONE',  ( 12.88139461472923841, -9.891864711284155121, 3.747395293195558847E-16 ) ) ;
#9700=CARTESIAN_POINT ( 'NONE',  ( 3.343943643650761022, -10.41127694127790271, 10.00000000000000000 ) ) ;
#9701=CARTESIAN_POINT ( 'NONE',  ( -8.211874628637438889, -10.69266484962706087, 6.857782953271941950E-17 ) ) ;
#9705=AXIS2_PLACEMENT_3D ( 'NONE', #9547, #2757, #2942 ) ;
#9711=CARTESIAN_POINT ( 'NONE',  ( 9.962304844536467030, 3.945508033568876360, 3.747395293195558847E-16 ) ) ;
#9715=ORIENTED_EDGE ( 'NONE', *, *, #6284, .F. ) ;
#9717=CARTESIAN_POINT ( 'NONE',  ( -12.06849956494803600, -5.462025159505909500, 10.00000000000000000 ) ) ;
#9728=CARTESIAN_POINT ( 'NONE',  ( 5.027256439335598515, -9.798587832408038878, 6.857782953271941950E-17 ) ) ;
#9735=CARTESIAN_POINT ( 'NONE',  ( -7.402161455537875412, -5.702533393948235663, 10.00000000000000000 ) ) ;
#9737=SURFACE_STYLE_FILL_AREA ( #10663 ) ;
#9741=CARTESIAN_POINT ( 'NONE',  ( 10.63538685525201188, -4.008487272325480966, 10.00000000000000000 ) ) ;
#9743=CARTESIAN_POINT ( 'NONE',  ( 16.25531780653859215, -2.690316503436295914, 3.747395293195558847E-16 ) ) ;
#9755=CARTESIAN_POINT ( 'NONE',  ( -5.965338750500730924, 7.524205049158505965, 10.00000000000000000 ) ) ;
#9757=CARTESIAN_POINT ( 'NONE',  ( -10.84705874452746066, 6.751620637727320684, 6.857782953271941950E-17 ) ) ;
#9760=ORIENTED_EDGE ( 'NONE', *, *, #6357, .F. ) ;
#9768=CARTESIAN_POINT ( 'NONE',  ( 10.50580257846853982, 1.391709641844861123, 3.747395293195558847E-16 ) ) ;
#9775=CARTESIAN_POINT ( 'NONE',  ( 13.06601448280975220, -5.920767845834314258, 10.00000000000000000 ) ) ;
#9780=UNCERTAINTY_MEASURE_WITH_UNIT (LENGTH_MEASURE( 1.000000000000000082E-05 ), #5031, 'distance_accuracy_value', 'NONE');
#9788=CARTESIAN_POINT ( 'NONE',  ( 7.252227276001472767, 5.017415995114415495, 6.857782953271941950E-17 ) ) ;
#9797=CARTESIAN_POINT ( 'NONE',  ( -12.04643853703213807, -0.2059847383341459892, 10.00000000000000000 ) ) ;
#9808=CARTESIAN_POINT ( 'NONE',  ( -8.665663522307777811, -5.581295667939715877, 10.00000000000000000 ) ) ;
#9810=CARTESIAN_POINT ( 'NONE',  ( 11.72652038055309731, 7.297668919379284524, 3.747395293195558847E-16 ) ) ;
#9822=CARTESIAN_POINT ( 'NONE',  ( 1.737537816361723220, -4.672682311025840640, 10.00000000000000000 ) ) ;
#9825=CARTESIAN_POINT ( 'NONE',  ( 5.835571643920552276, -9.386589068694823013, 6.857782953271941950E-17 ) ) ;
#9834=CARTESIAN_POINT ( 'NONE',  ( 2.839002905302877799, -15.63284973865751049, 10.00000000000000000 ) ) ;
#9840=CARTESIAN_POINT ( 'NONE',  ( 5.211919109253432936, 5.981019939437269173, 3.747395293195558847E-16 ) ) ;
#9846=CARTESIAN_POINT ( 'NONE',  ( 4.451863640886955409, 11.26298505921346305, 10.00000000000000000 ) ) ;
#9857=CARTESIAN_POINT ( 'NONE',  ( -7.130211940009568927, -7.605417807865418212, 6.857782953271941950E-17 ) ) ;
#9862=CARTESIAN_POINT ( 'NONE',  ( -5.008276813248565773, -11.55791719732261669, 10.00000000000000000 ) ) ;
#9869=CARTESIAN_POINT ( 'NONE',  ( 7.605204090344414247, 4.385345779697003010, 10.00000000000000000 ) ) ;
#9871=CARTESIAN_POINT ( 'NONE',  ( -11.32214898804403802, 3.633524203738173419, 3.747395293195558847E-16 ) ) ;
#9882=CARTESIAN_POINT ( 'NONE',  ( -4.859750766525547050, 4.557676925202722273, 10.00000000000000000 ) ) ;
#9884=CARTESIAN_POINT ( 'NONE',  ( -8.799721882313772170, 9.100398320382241835, 6.857782953271941950E-17 ) ) ;
#9885=SURFACE_STYLE_FILL_AREA ( #10807 ) ;
#9892=CARTESIAN_POINT ( 'NONE',  ( 7.983652613117085295, -10.39416588708253997, 10.00000000000000000 ) ) ;
#9895=CARTESIAN_POINT ( 'NONE',  ( -5.319913005755192437, -3.351504787100450855, 3.747395293195558847E-16 ) ) ;
#9901=CARTESIAN_POINT ( 'NONE',  ( -12.27443204882852257, 3.949650873796767492, 10.00000000000000000 ) ) ;
#9903=CARTESIAN_POINT ( 'NONE',  ( 4.525508228541173850, -0.2388087992699347017, 10.00000000000000000 ) ) ;
#9911=CARTESIAN_POINT ( 'NONE',  ( -6.506554845699739076, -8.196137552275128968, 6.857782953271941950E-17 ) ) ;
#9916=CARTESIAN_POINT ( 'NONE',  ( -0.1586286459269548865, 8.284426055182342097, 10.00000000000000000 ) ) ;
#9922=CARTESIAN_POINT ( 'NONE',  ( 10.96671743108979058, -3.132869264233008266, 10.00000000000000000 ) ) ;
#9924=CARTESIAN_POINT ( 'NONE',  ( 9.683839015878911383, 10.01260560230520547, 3.747395293195558847E-16 ) ) ;
#9936=CARTESIAN_POINT ( 'NONE',  ( 11.50231346626665285, 1.508968394323198847, 6.857782953271941950E-17 ) ) ;
#9946=CARTESIAN_POINT ( 'NONE',  ( -11.15100792855599110, -5.055838994807845488, 10.00000000000000000 ) ) ;
#9952=CARTESIAN_POINT ( 'NONE',  ( -5.846204292276366843, 1.022993486932169516, 3.747395293195558847E-16 ) ) ;
#9960=CARTESIAN_POINT ( 'NONE',  ( 0.5697670706242778937, -3.781298318517896551, 10.00000000000000000 ) ) ;
#9967=CARTESIAN_POINT ( 'NONE',  ( 4.764169229608189227, 7.652272242164855243, 6.857782953271941950E-17 ) ) ;
#9977=CARTESIAN_POINT ( 'NONE',  ( 5.892341078160698409, -4.186101517074010125, 10.00000000000000000 ) ) ;
#9983=CARTESIAN_POINT ( 'NONE',  ( -3.909826107003197215, 8.641065831729468627, 10.00000000000000000 ) ) ;
#9991=CARTESIAN_POINT ( 'NONE',  ( -4.491015865170908228, 3.510096388331549910, 3.747395293195558847E-16 ) ) ;
#9998=CARTESIAN_POINT ( 'NONE',  ( 0.0002901587068752367257, -4.749354241797645315, 10.00000000000000000 ) ) ;
#9999=CARTESIAN_POINT ( 'NONE',  ( 4.451863640887384399, 11.26298505921345594, 6.857782953271941950E-17 ) ) ;
#10006=CARTESIAN_POINT ( 'NONE',  ( 13.03626601087043113, 4.193914020169875911, 10.00000000000000000 ) ) ;
#10009=DIRECTION ( 'NONE',  ( -0.07332096784667033185, -0.9973083954695395326, 0.000000000000000000 ) ) ;
#10010=CARTESIAN_POINT ( 'NONE',  ( -2.214925388403154116, 4.996014981202573146, 3.747395293195558847E-16 ) ) ;
#10019=CARTESIAN_POINT ( 'NONE',  ( -0.4771094043438766641, 5.286185534804332065, 10.00000000000000000 ) ) ;
#10028=CARTESIAN_POINT ( 'NONE',  ( 8.539395351299290837, 0.2748098766782898217, 6.857782953271941950E-17 ) ) ;
#10037=CARTESIAN_POINT ( 'NONE',  ( -8.111627617515260624, 3.498804908652024093, 10.00000000000000000 ) ) ;
#10044=CARTESIAN_POINT ( 'NONE',  ( -3.764233030011072678, -6.516208816467838894, 10.00000000000000000 ) ) ;
#10054=CARTESIAN_POINT ( 'NONE',  ( -3.231136241382283725, -5.666136714102345984, 3.747395293195558847E-16 ) ) ;
#10060=CARTESIAN_POINT ( 'NONE',  ( 4.698850784960275639, -6.565226861933597391, 10.00000000000000000 ) ) ;
#10062=CARTESIAN_POINT ( 'NONE',  ( -1.032305814202111760, 6.265050879046235366, 6.857782953271941950E-17 ) ) ;
#10069=CARTESIAN_POINT ( 'NONE',  ( 13.53515989517831919, -0.2218654272303337005, 10.00000000000000000 ) ) ;
#10073=CARTESIAN_POINT ( 'NONE',  ( -0.7379871813790714885, -6.677365878963852808, 3.747395293195558847E-16 ) ) ;
#10079=CARTESIAN_POINT ( 'NONE',  ( 3.006682760306614632, 4.002877712838978752, 10.00000000000000000 ) ) ;
#10086=CARTESIAN_POINT ( 'NONE',  ( -6.947552178111042309, -1.615339808524891563, 6.857782953271941950E-17 ) ) ;
#10092=CARTESIAN_POINT ( 'NONE',  ( -1.515734900794040829, 8.225284064336937817, 10.00000000000000000 ) ) ;
#10101=CARTESIAN_POINT ( 'NONE',  ( 5.508953106497951779, 1.454581011951755043, 10.00000000000000000 ) ) ;
#10109=CARTESIAN_POINT ( 'NONE',  ( 16.46093749971205966, -1.349437486485980386, 10.00000000000000000 ) ) ;
#10114=CARTESIAN_POINT ( 'NONE',  ( -11.98007164540817371, 10.17225797950328214, 10.00000000000000000 ) ) ;
#10115=CARTESIAN_POINT ( 'NONE',  ( 3.666996827460249797, 4.772409917195337137, 6.857782953271941950E-17 ) ) ;
#10124=CARTESIAN_POINT ( 'NONE',  ( -3.516813791735897254, 7.717845097288996037, 10.00000000000000000 ) ) ;
#10127=CARTESIAN_POINT ( 'NONE',  ( -4.158289900079266133, 7.437556212723415605, 3.747395293195558847E-16 ) ) ;
#10156=CARTESIAN_POINT ( 'NONE',  ( -4.428608208598376450, -4.627450663479480752, 10.00000000000000000 ) ) ;
#10164=CARTESIAN_POINT ( 'NONE',  ( 4.503282398431824873, -2.806195971666264111, 10.00000000000000000 ) ) ;
#10174=CARTESIAN_POINT ( 'NONE',  ( 5.498207398720008854, -4.630339417915828371, 3.747395293195558847E-16 ) ) ;
#10181=CARTESIAN_POINT ( 'NONE',  ( 11.73504485001147835, -12.52947377801879192, 10.00000000000000000 ) ) ;
#10182=CARTESIAN_POINT ( 'NONE',  ( 4.503282398433332112, -2.806195971666638922, 6.857782953271941950E-17 ) ) ;
#10192=CARTESIAN_POINT ( 'NONE',  ( -8.799590028668788477, 7.703979956833879150, 10.00000000000000000 ) ) ;
#10197=CARTESIAN_POINT ( 'NONE',  ( 2.355103038863950893, 10.93470652055903791, 3.747395293195558847E-16 ) ) ;
#10215=CARTESIAN_POINT ( 'NONE',  ( 13.68367311611256554, -8.822018488634762790, 3.747395293195558847E-16 ) ) ;
#10216=CARTESIAN_POINT ( 'NONE',  ( -0.8869411547437818788, -7.669649013129171244, 6.857782953271941950E-17 ) ) ;
#10225=CARTESIAN_POINT ( 'NONE',  ( 3.006682760306614632, 4.002877712838978752, 10.00000000000000000 ) ) ;
#10230=CARTESIAN_POINT ( 'NONE',  ( -1.032305814202113092, 6.265050879046242471, 10.00000000000000000 ) ) ;
#10238=CARTESIAN_POINT ( 'NONE',  ( 7.402789038520869447, -0.9464297003978341394, 3.747395293195558847E-16 ) ) ;
#10245=CARTESIAN_POINT ( 'NONE',  ( -16.00307013876015461, -1.840746716621879830, 10.00000000000000000 ) ) ;
#10246=CARTESIAN_POINT ( 'NONE',  ( 1.661435237661581521, -7.700870200009177324, 6.857782953271941950E-17 ) ) ;
#10255=CARTESIAN_POINT ( 'NONE',  ( 9.962304844536470583, 3.945508033568877249, 10.00000000000000000 ) ) ;
#10260=CARTESIAN_POINT ( 'NONE',  ( -5.868204859621548586, -7.421994279450896848, 3.747395293195558847E-16 ) ) ;
#10269=DIRECTION ( 'NONE',  ( 3.061616997868383141E-16, -1.128098818916242718E-15, 1.000000000000000000 ) ) ;
#10271=CARTESIAN_POINT ( 'NONE',  ( 15.52845182490561271, -5.270724383582042094, 3.747395293195558847E-16 ) ) ;
#10272=CARTESIAN_POINT ( 'NONE',  ( 3.534825977509324257, -7.171832907601985774, 6.857782953271941950E-17 ) ) ;
#10287=CARTESIAN_POINT ( 'NONE',  ( -4.859750766525547050, 4.557676925202722273, 10.00000000000000000 ) ) ;
#10296=CARTESIAN_POINT ( 'NONE',  ( 10.01890055165175042, -12.63311126014650121, 10.00000000000000000 ) ) ;
#10301=CARTESIAN_POINT ( 'NONE',  ( -12.80690425020244128, 9.177692349400032867, 10.00000000000000000 ) ) ;
#10302=CARTESIAN_POINT ( 'NONE',  ( -4.859750766526011567, 4.557676925202717833, 6.857782953271941950E-17 ) ) ;
#10309=CARTESIAN_POINT ( 'NONE',  ( -0.1586286459269548865, 8.284426055182342097, 10.00000000000000000 ) ) ;
#10310=B_SPLINE_SURFACE_WITH_KNOTS ( 'NONE', 1, 3, ( 
 ( #9266, #9200, #942, #1796, #3639, #7293, #7355, #10181, #3697, #2780, #4677, #885, #5724, #6566, #3763, #1919, #3580, #8412, #8226, #11229, #6509, #11, #11046, #2657, #8481, #10245, #5594, #7484, #2842, #9448, #6390, #10301, #10114, #5655, #3822, #1008, #4742, #78, #7542, #11287, #2902, #6803, #5897, #11464, #3204, #9628, #2222, #317, #1249, #3138, #6923, #7727, #191, #1300, #8534, #7668, #5959, #10424, #131, #3029, #10539, #2044, #4055, #377, #10667, #7787, #10606, #1069, #5782, #9686, #5035, #6686, #4982, #2967, #6012, #11587, #6863, #11519, #3944, #2158, #8716, #2099, #2278, #8773, #9504, #4116, #1121, #7851, #5838, #4854, #4798, #10483, #8594, #3878, #11406, #6746, #259, #1178, #7599, #9566, #11342, #4920, #8660, #4001, #3085, #9922, #9741, #4356, #5154, #2458, #1359, #4181, #11874, #439, #10967, #558, #9009, #3445, #2399, #498, #1539, #7909, #4417, #5216, #9808, #4292, #11640, #6256, #5276, #5091, #8092, #8024, #11761, #3386, #7098, #5344, #6140, #3258, #9983, #6977, #10722, #3506, #10789, #11820, #1608, #2338, #1422, #10849, #2520, #625, #9869, #8836, #6073, #8893, #7218, #4236, #2590, #6197, #7155, #10903, #1481, #7962, #9074, #11696, #8149, #8947, #3316, #685, #7038, #2830, #1846, #10044, #926, #9253, #872, #8337, #3680, #1905, #2701, #9128, #6553, #11934, #7279, #63, #7339, #4663, #10287, #4474, #6378, #4606, #11215, #10230, #6436, #5400, #5638, #5521, #11086, #7404, #10101, #3809, #7529, #10164, #1665, #5581, #9371, #8210, #11148, #1779 ),
 ( #3567, #739, #989, #4730, #2762, #12058, #11030, #9181, #5452, #2644, #8467, #1718, #803, #11273, #5493, #6494, #9313, #7467, #8397, #4546, #6324, #3744, #8277, #12002, #3624, #9434, #2143, #2027, #9614, #6848, #5821, #1288, #4101, #5705, #7715, #6786, #5883, #305, #8759, #4043, #6610, #10592, #244, #10409, #11327, #11450, #2886, #7767, #3924, #5023, #10344, #4839, #2948, #1963, #11505, #10524, #5946, #7649, #1231, #8641, #11392, #6732, #1053, #1165, #5765, #3013, #359, #8705, #4968, #9490, #3988, #3069, #10466, #7834, #3128, #8521, #2205, #7584, #9673, #2085, #120, #4782, #177, #1107, #3863, #6670, #8578, #9551, #4904, #4279, #3242, #9059, #1525, #10835, #8994, #6910, #11746, #11571, #6185, #6963, #8007, #3191, #6000, #1591, #2266, #671, #2383, #2445, #5259, #4222, #2322, #3370, #9728, #6242, #7023, #11627, #6123, #1344, #8076, #7082, #10653, #9911, #9857, #1467, #5202, #8937, #7143, #7950, #5076, #11805, #8819, #424, #5326, #485, #608, #3435, #4169, #10707, #543, #4342, #10893, #11680, #7895, #2504, #10770, #3299, #9967, #6059, #4401, #9788, #1408, #5141, #8881, #7453, #10028, #857, #8258, #724, #12043, #3727, #1764, #4590, #6418, #10272, #8322, #9297, #7384, #3664, #10216, #1890, #2684, #7261, #8382, #3492, #2629, #914, #5387, #7202, #10086, #5505, #9114, #11127, #11200, #5624, #2747, #5567, #8136, #4460, #4647, #12100, #1653, #6478, #8195, #971, #3550, #10950, #11919, #6363, #7321, #11984, #1831, #11018, #9354, #2816, #6540, #11861, #2570, #6307 ) ),
 .UNSPECIFIED., .F., .F., .F.,
 ( 2, 2 ),
 ( 4, 2, 2, 2, 2, 2, 2, 2, 2, 2, 2, 2, 2, 2, 2, 2, 2, 2, 2, 2, 2, 2, 2, 2, 2, 2, 2, 2, 2, 2, 2, 2, 2, 2, 2, 2, 2, 2, 2, 2, 2, 2, 2, 2, 2, 2, 2, 2, 2, 2, 2, 2, 2, 2, 2, 2, 2, 2, 2, 2, 2, 2, 2, 2, 2, 2, 2, 2, 2, 2, 2, 2, 2, 2, 2, 2, 2, 2, 2, 2, 2, 2, 2, 2, 2, 2, 2, 2, 2, 2, 2, 2, 2, 2, 2, 2, 2, 2, 2, 2, 2, 2, 2, 4 ),
 ( 0.000000000000000000, 0.4545454545454546968 ),
 ( 0.000000000000000000, 0.007812500000000000000, 0.01562500000000000000, 0.02343750000000000000, 0.03125000000000000000, 0.03906250000000000000, 0.04687500000000000000, 0.05468750000000000000, 0.06250000000000000000, 0.07031250000000000000, 0.07812500000000000000, 0.08593750000000000000, 0.09375000000000000000, 0.1015625000000000000, 0.1093750000000000000, 0.1171875000000000000, 0.1250000000000000000, 0.1328125000000000000, 0.1406250000000000000, 0.1484375000000000000, 0.1562500000000000000, 0.1640625000000000000, 0.1718750000000000000, 0.1796875000000000000, 0.1875000000000000000, 0.1953125000000000000, 0.2031250000000000000, 0.2109375000000000000, 0.2187500000000000000, 0.2265625000000000000, 0.2343750000000000000, 0.2421875000000000000, 0.2500000000000000000, 0.2578125000000000000, 0.2656250000000000000, 0.2734375000000000000, 0.2812500000000000000, 0.2890625000000000000, 0.2968750000000000000, 0.3046875000000000000, 0.3125000000000000000, 0.3203125000000000000, 0.3281250000000000000, 0.3359375000000000000, 0.3437500000000000000, 0.3515625000000000000, 0.3593750000000000000, 0.3671875000000000000, 0.3750000000000000000, 0.3828125000000000000, 0.3906250000000000000, 0.3984375000000000000, 0.4062500000000000000, 0.4140625000000000000, 0.4218750000000000000, 0.4296875000000000000, 0.4375000000000000000, 0.4453125000000000000, 0.4531250000000000000, 0.4609375000000000000, 0.4687500000000000000, 0.4765625000000000000, 0.4843750000000000000, 0.4921875000000000000, 0.5000000000000000000, 0.5078125000000000000, 0.5156250000000000000, 0.5234375000000000000, 0.5312500000000000000, 0.5390625000000000000, 0.5468750000000000000, 0.5546875000000000000, 0.5625000000000000000, 0.5703125000000000000, 0.5781250000000000000, 0.5859375000000000000, 0.5937500000000000000, 0.6015625000000000000, 0.6093750000000000000, 0.6171875000000000000, 0.6250000000000000000, 0.6328125000000000000, 0.6406250000000000000, 0.6484375000000000000, 0.6562500000000000000, 0.6640625000000000000, 0.6718750000000000000, 0.6796875000000000000, 0.6875000000000000000, 0.6953125000000000000, 0.7031250000000000000, 0.7109375000000000000, 0.7187500000000000000, 0.7265625000000000000, 0.7343750000000000000, 0.7421875000000000000, 0.7500000000000000000, 0.7656250000000000000, 0.7812500000000000000, 0.7968750000000000000, 0.8125000000000000000, 0.8281250000000000000, 0.8437500000000000000, 0.8499999999999999778 ),
 .UNSPECIFIED. ) ;
#10312=CARTESIAN_POINT ( 'NONE',  ( -8.799590028668786701, 7.703979956834778875, 3.747395293195558847E-16 ) ) ;
#10324=VECTOR ( 'NONE', #5805, 999.9999999999998863 ) ;
#10329=CARTESIAN_POINT ( 'NONE',  ( 1.629745903656676376, 14.14889381255349932, 3.747395293195558847E-16 ) ) ;
#10335=CARTESIAN_POINT ( 'NONE',  ( 17.24531215409499296, -2.853661713830125013, 10.00000000000000000 ) ) ;
#10337=CARTESIAN_POINT ( 'NONE',  ( 1.631735293711821022, 4.895207720155140940, 10.00000000000000000 ) ) ;
#10344=CARTESIAN_POINT ( 'NONE',  ( 14.27634331491212016, 3.322769473268863738, 6.857782953271941950E-17 ) ) ;
#10352=CARTESIAN_POINT ( 'NONE',  ( 4.977139221860650942, 13.21892491369670530, 10.00000000000000000 ) ) ;
#10355=APPLICATION_CONTEXT ( 'automotive_design' ) ;
#10371=CARTESIAN_POINT ( 'NONE',  ( -1.307086582043127443, 11.26718560147321568, 10.00000000000000000 ) ) ;
#10375=CARTESIAN_POINT ( 'NONE',  ( 10.50580257846853982, 1.391709641844861123, 3.747395293195558847E-16 ) ) ;
#10392=CARTESIAN_POINT ( 'NONE',  ( -10.19073739998278505, -11.62312336453203443, 3.747395293195558847E-16 ) ) ;
#10400=CARTESIAN_POINT ( 'NONE',  ( 15.92723891616543774, -6.911623607273383207, 10.00000000000000000 ) ) ;
#10402=CARTESIAN_POINT ( 'NONE',  ( 3.194803811556594653, -2.743189786380181072, 10.00000000000000000 ) ) ;
#10409=CARTESIAN_POINT ( 'NONE',  ( 7.525577113297162946, 13.03378399180780534, 6.857782953271941950E-17 ) ) ;
#10418=CARTESIAN_POINT ( 'NONE',  ( 10.44364468045616157, 9.157203537818526584, 10.00000000000000000 ) ) ;
#10420=CARTESIAN_POINT ( 'NONE',  ( 17.49999999999999645, 0.000000000000000000, 6.857782953271941950E-17 ) ) ;
#10424=CARTESIAN_POINT ( 'NONE',  ( 11.14370178440676007, -8.845034901279914763, 10.00000000000000000 ) ) ;
#10427=CARTESIAN_POINT ( 'NONE',  ( -3.562082835880472587, -15.28349083755603388, 3.747395293195558847E-16 ) ) ;
#10435=CARTESIAN_POINT ( 'NONE',  ( 5.657123057053187409, 5.504982807385219168, 10.00000000000000000 ) ) ;
#10438=CARTESIAN_POINT ( 'NONE',  ( 9.246005348854476225, -6.405614325510554430, 10.00000000000000000 ) ) ;
#10439=CARTESIAN_POINT ( 'NONE',  ( -14.76245309360481706, 5.834016798581969532, 6.857782953271941950E-17 ) ) ;
#10450=LINE ( 'NONE', #2067, #10324 ) ;
#10452=CARTESIAN_POINT ( 'NONE',  ( -4.054747718262373901, -11.96785467447665674, 3.747395293195558847E-16 ) ) ;
#10456=PRODUCT_CONTEXT ( 'NONE', #10355, 'mechanical' ) ;
#10460=CARTESIAN_POINT ( 'NONE',  ( 4.321204520403006732, 2.017656881711013206, 10.00000000000000000 ) ) ;
#10466=CARTESIAN_POINT ( 'NONE',  ( -10.47176928358604364, -8.303818807687074255, 6.857782953271941950E-17 ) ) ;
#10477=CARTESIAN_POINT ( 'NONE',  ( 12.15471013770155295, -5.500887282572486825, 10.00000000000000000 ) ) ;
#10483=CARTESIAN_POINT ( 'NONE',  ( 1.597090680284417807, 12.12373805211591460, 10.00000000000000000 ) ) ;
#10486=CARTESIAN_POINT ( 'NONE',  ( -3.043536693350106681, 14.07442491708025756, 3.747395293195558847E-16 ) ) ;
#10494=CARTESIAN_POINT ( 'NONE',  ( -5.846204292276370396, 1.022993486932170404, 10.00000000000000000 ) ) ;
#10496=CARTESIAN_POINT ( 'NONE',  ( 8.539395351299297943, 0.2748098766782894331, 10.00000000000000000 ) ) ;
#10497=CARTESIAN_POINT ( 'NONE',  ( -3.251399079312188078, 15.05603916236422180, 6.857782953271941950E-17 ) ) ;
#10504=CARTESIAN_POINT ( 'NONE',  ( 0.2749788638910972693, -16.81181333738675221, 6.857782953271941950E-17 ) ) ;
#10509=CARTESIAN_POINT ( 'NONE',  ( 9.640149279600553456, 4.768118462334743235, 3.747395293195558847E-16 ) ) ;
#10524=CARTESIAN_POINT ( 'NONE',  ( 13.06601448280974509, -5.920767845834311593, 6.857782953271941950E-17 ) ) ;
#10533=CARTESIAN_POINT ( 'NONE',  ( 9.623054350189521600, -9.012277985855607909, 10.00000000000000000 ) ) ;
#10539=CARTESIAN_POINT ( 'NONE',  ( 7.619603487155713673, -11.82824555707897218, 10.00000000000000000 ) ) ;
#10543=VECTOR ( 'NONE', #3362, 1000.000000000000000 ) ;
#10551=CARTESIAN_POINT ( 'NONE',  ( 4.212679447664378074, 6.814025269448781508, 10.00000000000000000 ) ) ;
#10554=CARTESIAN_POINT ( 'NONE',  ( 9.623984404418655103, 6.889883918979096578, 10.00000000000000000 ) ) ;
#10556=CARTESIAN_POINT ( 'NONE',  ( 2.259453438922057522, -13.68937604509904027, 6.857782953271941950E-17 ) ) ;
#10565=( GEOMETRIC_REPRESENTATION_CONTEXT ( 3 ) GLOBAL_UNCERTAINTY_ASSIGNED_CONTEXT ( ( #9780 ) ) GLOBAL_UNIT_ASSIGNED_CONTEXT ( ( #5031, #314, #1244 ) ) REPRESENTATION_CONTEXT ( 'NONE', 'WORKASPACE' ) );
#10566=CARTESIAN_POINT ( 'NONE',  ( 11.04976219204224996, -11.79656285005915350, 10.00000000000000000 ) ) ;
#10574=CARTESIAN_POINT ( 'NONE',  ( -10.00031051369627022, 6.213292778946845729, 3.747395293195558847E-16 ) ) ;
#10580=CARTESIAN_POINT ( 'NONE',  ( 0.5005346673319861495, 15.27733729710888255, 10.00000000000000000 ) ) ;
#10592=CARTESIAN_POINT ( 'NONE',  ( 4.165359127293307040, 14.58480927028732843, 6.857782953271941950E-17 ) ) ;
#10600=CARTESIAN_POINT ( 'NONE',  ( 2.355103038863951781, 10.93470652055904146, 10.00000000000000000 ) ) ;
#10606=CARTESIAN_POINT ( 'NONE',  ( -2.240087900411203758, -13.53314956822678639, 10.00000000000000000 ) ) ;
#10615=CARTESIAN_POINT ( 'NONE',  ( 16.50000000000000000, 0.000000000000000000, 3.747395293195558847E-16 ) ) ;
#10616=CARTESIAN_POINT ( 'NONE',  ( 7.261170810407329590, -1.543028577657542311, 10.00000000000000000 ) ) ;
#10621=CARTESIAN_POINT ( 'NONE',  ( 11.40744677810891083, -1.317628706759891966, 10.00000000000000000 ) ) ;
#10624=CARTESIAN_POINT ( 'NONE',  ( -12.80690425020131684, 9.177692349400029315, 6.857782953271941950E-17 ) ) ;
#10633=CARTESIAN_POINT ( 'NONE',  ( 4.123629756450001516, -15.38522696314584870, 10.00000000000000000 ) ) ;
#10638=CARTESIAN_POINT ( 'NONE',  ( -9.037587479195730467, -0.7561632655184011842, 3.747395293195558847E-16 ) ) ;
#10643=CARTESIAN_POINT ( 'NONE',  ( 14.22875512193219372, -2.589574901423981501, 10.00000000000000000 ) ) ;
#10653=CARTESIAN_POINT ( 'NONE',  ( -5.125696908148159814, -9.212757455309411370, 6.857782953271941950E-17 ) ) ;
#10660=CARTESIAN_POINT ( 'NONE',  ( -5.868204859621552139, -7.421994279450156107, 10.00000000000000000 ) ) ;
#10663=FILL_AREA_STYLE ('',( #9682 ) ) ;
#10667=CARTESIAN_POINT ( 'NONE',  ( 1.124919223378051392, -13.78906249641292270, 10.00000000000000000 ) ) ;
#10669=CARTESIAN_POINT ( 'NONE',  ( 16.46093749971205611, -1.349437486485979498, 3.747395293195558847E-16 ) ) ;
#10679=CARTESIAN_POINT ( 'NONE',  ( 7.737545192982512532, 9.111483571581279861, 10.00000000000000000 ) ) ;
#10680=CARTESIAN_POINT ( 'NONE',  ( -9.386162357322611172, -4.067606288967436257, 6.857782953271941950E-17 ) ) ;
#10690=CARTESIAN_POINT ( 'NONE',  ( 4.071483724746831179, 10.33449570568845033, 3.747395293195558847E-16 ) ) ;
#10696=( NAMED_UNIT ( * ) SI_UNIT ( $, .STERADIAN. ) SOLID_ANGLE_UNIT ( ) );
#10697=CARTESIAN_POINT ( 'NONE',  ( -4.389456771235332511, 11.66511648340389762, 10.00000000000000000 ) ) ;
#10707=CARTESIAN_POINT ( 'NONE',  ( -4.625218816436122538, 8.325684435358754243, 6.857782953271941950E-17 ) ) ;
#10714=CARTESIAN_POINT ( 'NONE',  ( 6.391761267591818729, 8.940137919804724831, 10.00000000000000000 ) ) ;
#10717=PRESENTATION_STYLE_ASSIGNMENT (( #6973 ) ) ;
#10722=CARTESIAN_POINT ( 'NONE',  ( -1.672018190274039418, 9.216430685901391584, 10.00000000000000000 ) ) ;
#10725=CARTESIAN_POINT ( 'NONE',  ( -7.594692469639082510, -9.901549393537251831, 3.747395293195558847E-16 ) ) ;
#10736=CARTESIAN_POINT ( 'NONE',  ( -5.248573321596930796, 4.168074790661433049, 10.00000000000000000 ) ) ;
#10739=CARTESIAN_POINT ( 'NONE',  ( -9.960937504979705537, 0.8181230654449899165, 6.857782953271941950E-17 ) ) ;
#10749=CARTESIAN_POINT ( 'NONE',  ( -5.359287035703753865, 6.724520318540387009, 3.747395293195558847E-16 ) ) ;
#10757=CARTESIAN_POINT ( 'NONE',  ( -1.410059164928063380, 12.26527237696110184, 10.00000000000000000 ) ) ;
#10770=CARTESIAN_POINT ( 'NONE',  ( 2.798030692818294085, 8.692477993603722197, 6.857782953271941950E-17 ) ) ;
#10779=CARTESIAN_POINT ( 'NONE',  ( 10.39479819782869896, 2.258419626871297492, 10.00000000000000000 ) ) ;
#10789=CARTESIAN_POINT ( 'NONE',  ( 0.6097887191948987429, 9.229167205757272896, 10.00000000000000000 ) ) ;
#10791=CARTESIAN_POINT ( 'NONE',  ( -9.680665087125342794, -7.686621967951971612, 3.747395293195558847E-16 ) ) ;
#10799=DIRECTION ( 'NONE',  ( -1.000000000000000000, 0.000000000000000000, 3.061616997868383141E-16 ) ) ;
#10804=CARTESIAN_POINT ( 'NONE',  ( -7.040021908109685533, -0.4595208068205508534, 10.00000000000000000 ) ) ;
#10806=CARTESIAN_POINT ( 'NONE',  ( -11.39998097177137026, 5.856612080558655897, 6.857782953271941950E-17 ) ) ;
#10807=FILL_AREA_STYLE ('',( #7054 ) ) ;
#10814=CARTESIAN_POINT ( 'NONE',  ( -14.61026919807147451, 3.159152207411757285, 10.00000000000000000 ) ) ;
#10820=CARTESIAN_POINT ( 'NONE',  ( 4.212679447664376298, 6.814025269448777955, 3.747395293195558847E-16 ) ) ;
#10825=CARTESIAN_POINT ( 'NONE',  ( -10.84705874452746777, 6.751620637726422736, 10.00000000000000000 ) ) ;
#10827=CARTESIAN_POINT ( 'NONE',  ( 0.07364157424580680678, -3.751631698233684364, 10.00000000000000000 ) ) ;
#10835=CARTESIAN_POINT ( 'NONE',  ( 4.451863640887384399, 11.26298505921345594, 6.857782953271941950E-17 ) ) ;
#10841=CARTESIAN_POINT ( 'NONE',  ( 9.640149279600557009, 4.768118462334745011, 10.00000000000000000 ) ) ;
#10849=CARTESIAN_POINT ( 'NONE',  ( 5.893263639827395650, 6.717612500730409941, 10.00000000000000000 ) ) ;
#10851=CARTESIAN_POINT ( 'NONE',  ( 11.62709622633471618, -6.461356448465071622, 3.747395293195558847E-16 ) ) ;
#10867=CARTESIAN_POINT ( 'NONE',  ( -2.764021070441483374, -10.29567250283335689, 6.857782953271941950E-17 ) ) ;
#10874=CARTESIAN_POINT ( 'NONE',  ( 5.172292865810427465, -11.91455349003027919, 10.00000000000000000 ) ) ;
#10877=CARTESIAN_POINT ( 'NONE',  ( -4.763935748648512991, -4.221771024091821367, 3.747395293195558847E-16 ) ) ;
#10885=CARTESIAN_POINT ( 'NONE',  ( 4.321204520403006732, 2.017656881711013206, 10.00000000000000000 ) ) ;
#10893=CARTESIAN_POINT ( 'NONE',  ( -1.672018190274121574, 9.216430685901386255, 6.857782953271941950E-17 ) ) ;
#10898=CARTESIAN_POINT ( 'NONE',  ( -5.319913005755715574, -3.351504787099933047, 10.00000000000000000 ) ) ;
#10903=CARTESIAN_POINT ( 'NONE',  ( 6.689389171169565884, -4.795626085247176817, 10.00000000000000000 ) ) ;
#10910=CARTESIAN_POINT ( 'NONE',  ( 4.321204520403003180, 2.017656881711011430, 3.747395293195558847E-16 ) ) ;
#10917=CARTESIAN_POINT ( 'NONE',  ( -2.570438583093578533, 5.934334910739571534, 10.00000000000000000 ) ) ;
#10918=CARTESIAN_POINT ( 'NONE',  ( -0.1814876354083659327, -10.77628937513454943, 6.857782953271941950E-17 ) ) ;
#10927=CARTESIAN_POINT ( 'NONE',  ( -11.99326810842507562, 8.590522060507204571, 10.00000000000000000 ) ) ;
#10933=CARTESIAN_POINT ( 'NONE',  ( -0.1881845630465192321, -6.755137126427047001, 3.747395293195558847E-16 ) ) ;
#10950=CARTESIAN_POINT ( 'NONE',  ( 3.666996827460249797, 4.772409917195337137, 6.857782953271941950E-17 ) ) ;
#10959=CARTESIAN_POINT ( 'NONE',  ( -5.862605222286289219, -1.923479314576678423, 10.00000000000000000 ) ) ;
#10963=( GEOMETRIC_REPRESENTATION_CONTEXT ( 3 ) GLOBAL_UNCERTAINTY_ASSIGNED_CONTEXT ( ( #852 ) ) GLOBAL_UNIT_ASSIGNED_CONTEXT ( ( #3873, #7480, #10696 ) ) REPRESENTATION_CONTEXT ( 'NONE', 'WORKASPACE' ) );
#10967=CARTESIAN_POINT ( 'NONE',  ( 2.469054641153702434, -10.61194774715159994, 10.00000000000000000 ) ) ;
#10976=CARTESIAN_POINT ( 'NONE',  ( -1.784247137544765716, 5.123456263349895679, 3.747395293195558847E-16 ) ) ;
#10985=CARTESIAN_POINT ( 'NONE',  ( -6.191802569540381995, -3.848120238388911041, 10.00000000000000000 ) ) ;
#10986=CARTESIAN_POINT ( 'NONE',  ( 5.531377455021717182, -0.3672033614207537711, 6.857782953271941950E-17 ) ) ;
#10993=ORIENTED_EDGE ( 'NONE', *, *, #5608, .F. ) ;
#10995=CARTESIAN_POINT ( 'NONE',  ( -3.043536693350107569, 14.07442491708026111, 10.00000000000000000 ) ) ;
#11001=CARTESIAN_POINT ( 'NONE',  ( 5.657123057053811799, 5.504982807385217392, 3.747395293195558847E-16 ) ) ;
#11010=CARTESIAN_POINT ( 'NONE',  ( -0.9167995209625440234, 5.268308710424125074, 10.00000000000000000 ) ) ;
#11018=CARTESIAN_POINT ( 'NONE',  ( 4.503282398433332112, -2.806195971666638922, 6.857782953271941950E-17 ) ) ;
#11024=CARTESIAN_POINT ( 'NONE',  ( -5.704017324792772570, 1.489539271746576743, 10.00000000000000000 ) ) ;
#11030=CARTESIAN_POINT ( 'NONE',  ( 13.67726327739689829, -10.50289975150003485, 6.857782953271941950E-17 ) ) ;
#11039=CARTESIAN_POINT ( 'NONE',  ( 16.50000000000000355, 0.000000000000000000, 10.00000000000000000 ) ) ;
#11046=CARTESIAN_POINT ( 'NONE',  ( -14.12277927129996158, -8.146689865454478152, 10.00000000000000000 ) ) ;
#11047=CARTESIAN_POINT ( 'NONE',  ( 5.312937634499088624, -1.259815497212412261, 6.857782953271941950E-17 ) ) ;
#11052=CARTESIAN_POINT ( 'NONE',  ( 13.24268851590354146, -2.403973981685017414, 10.00000000000000000 ) ) ;
#11056=CARTESIAN_POINT ( 'NONE',  ( 2.084958754360775934, -3.480815169281481047, 3.747395293195558847E-16 ) ) ;
#11079=CARTESIAN_POINT ( 'NONE',  ( -5.962113107391272315, -1.426310550302921865, 10.00000000000000000 ) ) ;
#11086=CARTESIAN_POINT ( 'NONE',  ( 4.346347989804005607, 4.041826679702273495, 10.00000000000000000 ) ) ;
#11093=CARTESIAN_POINT ( 'NONE',  ( -4.763935748648512991, -4.221771024091821367, 3.747395293195558847E-16 ) ) ;
#11101=CARTESIAN_POINT ( 'NONE',  ( 8.235329212250112718, -1.783486464602660027, 6.857782953271941950E-17 ) ) ;
#11109=CARTESIAN_POINT ( 'NONE',  ( 7.316052646047090491, -7.060001943526881263, 10.00000000000000000 ) ) ;
#11112=CARTESIAN_POINT ( 'NONE',  ( 3.656769781543557141, 7.172433557890304456, 3.747395293195558847E-16 ) ) ;
#11124=FACE_OUTER_BOUND ( 'NONE', #19, .T. ) ;
#11126=CARTESIAN_POINT ( 'NONE',  ( 13.03626601087042758, 4.193914020170396384, 3.747395293195558847E-16 ) ) ;
#11127=CARTESIAN_POINT ( 'NONE',  ( -6.825012239887737309, 1.243808647927286515, 6.857782953271941950E-17 ) ) ;
#11137=CARTESIAN_POINT ( 'NONE',  ( 6.411932913581408044, 4.469049885107577502, 10.00000000000000000 ) ) ;
#11148=CARTESIAN_POINT ( 'NONE',  ( 0.3111040546027374343, -4.780743156735979049, 10.00000000000000000 ) ) ;
#11159=CARTESIAN_POINT ( 'NONE',  ( -3.038216613429991053, 4.635879136410029133, 3.747395293195558847E-16 ) ) ;
#11167=FACE_OUTER_BOUND ( 'NONE', #8815, .T. ) ;
#11168=CARTESIAN_POINT ( 'NONE',  ( 8.393308867179008814, -1.106660293010312213, 6.857782953271941950E-17 ) ) ;
#11179=CARTESIAN_POINT ( 'NONE',  ( 5.319643049700913728, -8.526005966359200272, 10.00000000000000000 ) ) ;
#11183=CARTESIAN_POINT ( 'NONE',  ( 4.071483724746831179, 10.33449570568845033, 3.747395293195558847E-16 ) ) ;
#11199=CARTESIAN_POINT ( 'NONE',  ( -11.21689850597007343, 9.520844388990626683, 3.747395293195558847E-16 ) ) ;
#11200=CARTESIAN_POINT ( 'NONE',  ( -6.661525743073264394, 1.789546221321740793, 6.857782953271941950E-17 ) ) ;
#11204=COLOUR_RGB ( '', 0.40784314, 0.44705882, 0.49803922) ;
#11208=CARTESIAN_POINT ( 'NONE',  ( 3.678979105947490780, -2.215585777442456550, 10.00000000000000000 ) ) ;
#11215=CARTESIAN_POINT ( 'NONE',  ( -2.061894914253513456, 6.087690860853038899, 10.00000000000000000 ) ) ;
#11222=CARTESIAN_POINT ( 'NONE',  ( 0.2599977045011495624, -15.80854529698373945, 10.00000000000000000 ) ) ;
#11229=CARTESIAN_POINT ( 'NONE',  ( -10.85385039129053197, -12.37615246896657872, 10.00000000000000000 ) ) ;
#11231=CARTESIAN_POINT ( 'NONE',  ( 7.449730884303669143, -3.679036338562942543, 6.857782953271941950E-17 ) ) ;
#11241=CARTESIAN_POINT ( 'NONE',  ( 10.51453309316909568, -0.3307463982597985686, 10.00000000000000000 ) ) ;
#11242=CARTESIAN_POINT ( 'NONE',  ( 17.50000000000000000, 0.000000000000000000, 10.00000000000000000 ) ) ;
#11243=CARTESIAN_POINT ( 'NONE',  ( -8.111627617515257072, 3.498804908652022316, 3.747395293195558847E-16 ) ) ;
#11258=CARTESIAN_POINT ( 'NONE',  ( 16.46093749971205611, -1.349437486485979498, 3.747395293195558847E-16 ) ) ;
#11272=CARTESIAN_POINT ( 'NONE',  ( 16.50000000000000355, 0.000000000000000000, 10.00000000000000000 ) ) ;
#11273=CARTESIAN_POINT ( 'NONE',  ( 0.2749788638910972693, -16.81181333738675221, 6.857782953271941950E-17 ) ) ;
#11282=CARTESIAN_POINT ( 'NONE',  ( -3.562082835880472587, -15.28349083755603743, 10.00000000000000000 ) ) ;
#11287=CARTESIAN_POINT ( 'NONE',  ( 0.5005346673319861495, 15.27733729710888255, 10.00000000000000000 ) ) ;
#11295=CARTESIAN_POINT ( 'NONE',  ( -5.868204859621552139, -7.421994279450156107, 10.00000000000000000 ) ) ;
#11299=CARTESIAN_POINT ( 'NONE',  ( -10.00031051369627022, 6.213292778946845729, 3.747395293195558847E-16 ) ) ;
#11313=CARTESIAN_POINT ( 'NONE',  ( -3.562082835880472587, -15.28349083755603388, 3.747395293195558847E-16 ) ) ;
#11322=FACE_OUTER_BOUND ( 'NONE', #7179, .T. ) ;
#11327=CARTESIAN_POINT ( 'NONE',  ( 8.547432504762587868, 12.33942397201039753, 6.857782953271941950E-17 ) ) ;
#11335=CARTESIAN_POINT ( 'NONE',  ( 7.019749797092301513, 12.16723183298456057, 10.00000000000000000 ) ) ;
#11342=CARTESIAN_POINT ( 'NONE',  ( 10.90031251054716499, 4.301772984117411269, 10.00000000000000000 ) ) ;
#11353=CARTESIAN_POINT ( 'NONE',  ( -5.359287035704432434, 6.724520318541068242, 10.00000000000000000 ) ) ;
#11356=CARTESIAN_POINT ( 'NONE',  ( 5.835571643920557605, -9.386589068694828342, 10.00000000000000000 ) ) ;
#11357=CARTESIAN_POINT ( 'NONE',  ( 10.35108484788238670, -9.702746953904560101, 6.857782953271941950E-17 ) ) ;
#11374=CARTESIAN_POINT ( 'NONE',  ( 7.019749797092834420, 12.16723183298349120, 3.747395293195558847E-16 ) ) ;
#11383=CARTESIAN_POINT ( 'NONE',  ( 8.281812197879521165, -14.90260015151097228, 10.00000000000000000 ) ) ;
#11392=CARTESIAN_POINT ( 'NONE',  ( 7.619603487155711008, -11.82824555707797387, 6.857782953271941950E-17 ) ) ;
#11401=CARTESIAN_POINT ( 'NONE',  ( 12.96212312671954514, -3.473279994529783199, 10.00000000000000000 ) ) ;
#11406=CARTESIAN_POINT ( 'NONE',  ( 5.343773788080183884, 10.82393792025544421, 10.00000000000000000 ) ) ;
#11410=CARTESIAN_POINT ( 'NONE',  ( 0.2599977045009999599, -15.80854529698373589, 3.747395293195558847E-16 ) ) ;
#11419=CARTESIAN_POINT ( 'NONE',  ( 7.357672848543034050, 2.125097602832379806, 10.00000000000000000 ) ) ;
#11421=CARTESIAN_POINT ( 'NONE',  ( -9.386162357322616501, -4.067606288967439809, 10.00000000000000000 ) ) ;
#11422=CARTESIAN_POINT ( 'NONE',  ( -10.11701526667143725, 11.92482893257633414, 6.857782953271941950E-17 ) ) ;
#11433=CARTESIAN_POINT ( 'NONE',  ( -3.141381368648054284, 10.98006565327106188, 3.747395293195558847E-16 ) ) ;
#11450=CARTESIAN_POINT ( 'NONE',  ( 10.38524206949620243, 10.73010674553377264, 6.857782953271941950E-17 ) ) ;
#11458=CARTESIAN_POINT ( 'NONE',  ( 9.683839015878914935, 10.01260560230626595, 10.00000000000000000 ) ) ;
#11464=CARTESIAN_POINT ( 'NONE',  ( 7.525577113297165610, 13.03378399180780889, 10.00000000000000000 ) ) ;
#11466=CARTESIAN_POINT ( 'NONE',  ( -10.19073739998278505, -11.62312336453203443, 3.747395293195558847E-16 ) ) ;
#11474=CARTESIAN_POINT ( 'NONE',  ( -5.704017324792772570, 1.489539271746576743, 10.00000000000000000 ) ) ;
#11477=CARTESIAN_POINT ( 'NONE',  ( 10.54603994011899459, 5.199563424939650957, 10.00000000000000000 ) ) ;
#11478=CARTESIAN_POINT ( 'NONE',  ( -7.327987143158983585, -11.36402271042705614, 6.857782953271941950E-17 ) ) ;
#11485=CARTESIAN_POINT ( 'NONE',  ( 16.46093749971205966, -1.349437486485980386, 10.00000000000000000 ) ) ;
#11490=CARTESIAN_POINT ( 'NONE',  ( -2.069312577552832266, -12.54440658741723880, 3.747395293195558847E-16 ) ) ;
#11497=CARTESIAN_POINT ( 'NONE',  ( 10.64229886435067662, -13.41933351754326154, 6.857782953271941950E-17 ) ) ;
#11505=CARTESIAN_POINT ( 'NONE',  ( 13.92981926110967450, -3.738495919395730116, 6.857782953271941950E-17 ) ) ;
#11514=CARTESIAN_POINT ( 'NONE',  ( -7.594692469639083399, -9.901549393538205734, 10.00000000000000000 ) ) ;
#11519=CARTESIAN_POINT ( 'NONE',  ( -13.04979933117209967, -0.2127334381860513379, 10.00000000000000000 ) ) ;
#11533=CARTESIAN_POINT ( 'NONE',  ( -6.012500708481080203, 0.06204199954272103523, 10.00000000000000000 ) ) ;
#11537=CARTESIAN_POINT ( 'NONE',  ( -6.506554845699742629, -8.196137552274390004, 10.00000000000000000 ) ) ;
#11538=CARTESIAN_POINT ( 'NONE',  ( 13.99323099382916169, 4.495563823643927037, 6.857782953271941950E-17 ) ) ;
#11553=CARTESIAN_POINT ( 'NONE',  ( -8.457858257354885723, -3.686763380685289970, 3.747395293195558847E-16 ) ) ;
#11559=CARTESIAN_POINT ( 'NONE',  ( 10.38524206949726469, 10.73010674553377797, 10.00000000000000000 ) ) ;
#11571=CARTESIAN_POINT ( 'NONE',  ( 9.056240860197961595, 7.682302481599242228, 6.857782953271941950E-17 ) ) ;
#11580=CARTESIAN_POINT ( 'NONE',  ( -3.937910939466569005, -8.732312745279401156, 10.00000000000000000 ) ) ;
#11587=CARTESIAN_POINT ( 'NONE',  ( -12.72059027619867955, -3.407653011836159873, 10.00000000000000000 ) ) ;
#11593=ADVANCED_FACE ( 'NONE', ( #3012 ), #8019, .F. ) ;
#11594=STYLED_ITEM ( 'NONE', ( #3407 ), #4621 ) ;
#11599=CARTESIAN_POINT ( 'NONE',  ( -2.433178163897189883, 9.086443520544605690, 10.00000000000000000 ) ) ;
#11601=CARTESIAN_POINT ( 'NONE',  ( 1.124919223378051392, -13.78906249641291559, 6.857782953271941950E-17 ) ) ;
#11611=CARTESIAN_POINT ( 'NONE',  ( -6.430932688512553064, -6.885836206077581068, 3.747395293195558847E-16 ) ) ;
#11616=CARTESIAN_POINT ( 'NONE',  ( 12.50121531544689013, -6.953993600215019555, 10.00000000000000000 ) ) ;
#11627=CARTESIAN_POINT ( 'NONE',  ( 0.7062845326066684581, -10.79445016380498501, 6.857782953271941950E-17 ) ) ;
#11633=CARTESIAN_POINT ( 'NONE',  ( -11.98301361336074500, 0.7816210414391656647, 10.00000000000000000 ) ) ;
#11634=ORIENTED_EDGE ( 'NONE', *, *, #6898, .T. ) ;
#11640=CARTESIAN_POINT ( 'NONE',  ( -9.650762677556034674, -3.270672451565360461, 10.00000000000000000 ) ) ;
#11642=CARTESIAN_POINT ( 'NONE',  ( -1.872083171988683015, 14.23747171912756038, 3.747395293195558847E-16 ) ) ;
#11653=CARTESIAN_POINT ( 'NONE',  ( 6.242895496889244278, -5.302832405932367266, 10.00000000000000000 ) ) ;
#11654=CARTESIAN_POINT ( 'NONE',  ( -9.650762677556027569, -3.270672451565358685, 6.857782953271941950E-17 ) ) ;
#11660=CARTESIAN_POINT ( 'NONE',  ( 0.2599977045011495624, -15.80854529698373945, 10.00000000000000000 ) ) ;
#11664=CARTESIAN_POINT ( 'NONE',  ( 9.701579622837702033, -3.641351606116561612, 3.747395293195558847E-16 ) ) ;
#11670=CARTESIAN_POINT ( 'NONE',  ( -9.783806739528735363, -9.162509837619124298, 10.00000000000000000 ) ) ;
#11680=CARTESIAN_POINT ( 'NONE',  ( -0.1504880127286837288, 9.287785325659760005, 6.857782953271941950E-17 ) ) ;
#11688=CARTESIAN_POINT ( 'NONE',  ( -4.054747718262374789, -11.96785467447666029, 10.00000000000000000 ) ) ;
#11696=CARTESIAN_POINT ( 'NONE',  ( 3.534825977509327366, -7.171832907601992879, 10.00000000000000000 ) ) ;
#11698=CARTESIAN_POINT ( 'NONE',  ( -12.04643853703213452, -0.2059847383342608973, 3.747395293195558847E-16 ) ) ;
#11710=CARTESIAN_POINT ( 'NONE',  ( 4.503282398431824873, -2.806195971666264111, 10.00000000000000000 ) ) ;
#11712=CARTESIAN_POINT ( 'NONE',  ( -2.433178163897522506, 9.086443520544598584, 6.857782953271941950E-17 ) ) ;
#11720=CARTESIAN_POINT ( 'NONE',  ( 2.103398428914359908, -12.69820342197951035, 10.00000000000000000 ) ) ;
#11723=CARTESIAN_POINT ( 'NONE',  ( 7.536008357046521944, 0.2705779428718260160, 3.747395293195558847E-16 ) ) ;
#11731=COLOUR_RGB ( '', 0.40784314, 0.44705882, 0.49803922) ;
#11733=CARTESIAN_POINT ( 'NONE',  ( -4.384918567263696332, -12.91535881965571342, 10.00000000000000000 ) ) ;
#11746=CARTESIAN_POINT ( 'NONE',  ( 7.737545192982509867, 9.111483571581276308, 6.857782953271941950E-17 ) ) ;
#11753=CARTESIAN_POINT ( 'NONE',  ( 10.41236255589547177, -1.188820951657899361, 10.00000000000000000 ) ) ;
#11761=CARTESIAN_POINT ( 'NONE',  ( -9.023584016175229650, 3.917288190900558131, 10.00000000000000000 ) ) ;
#11763=CARTESIAN_POINT ( 'NONE',  ( 7.019749797092834420, 12.16723183298349120, 3.747395293195558847E-16 ) ) ;
#11776=CARTESIAN_POINT ( 'NONE',  ( 6.689389171169565884, -4.795626085247176817, 10.00000000000000000 ) ) ;
#11778=CARTESIAN_POINT ( 'NONE',  ( 9.246005348854470896, -6.405614325511344909, 6.857782953271941950E-17 ) ) ;
#11779=SURFACE_STYLE_USAGE ( .BOTH. , #8045 ) ;
#11787=CARTESIAN_POINT ( 'NONE',  ( 4.163410377374356486, -12.26152398776834396, 10.00000000000000000 ) ) ;
#11789=LINE ( 'NONE', #654, #8769 ) ;
#11790=CARTESIAN_POINT ( 'NONE',  ( 0.5199114366211738947, 8.229807867079655281, 3.747395293195558847E-16 ) ) ;
#11805=CARTESIAN_POINT ( 'NONE',  ( -9.960937504979705537, 0.8181230654449899165, 6.857782953271941950E-17 ) ) ;
#11811=CARTESIAN_POINT ( 'NONE',  ( 4.623190192904714557, -5.402202315098911356, 10.00000000000000000 ) ) ;
#11820=CARTESIAN_POINT ( 'NONE',  ( 2.084091085258986897, 8.931495281877387171, 10.00000000000000000 ) ) ;
#11822=CARTESIAN_POINT ( 'NONE',  ( 7.983652613117083519, -10.39416588708253819, 3.747395293195558847E-16 ) ) ;
#11828=CARTESIAN_POINT ( 'NONE',  ( 3.006682760306612856, 4.002877712838976976, 3.747395293195558847E-16 ) ) ;
#11833=CARTESIAN_POINT ( 'NONE',  ( 0.6279411196271856843, -4.781877258324073843, 10.00000000000000000 ) ) ;
#11836=CARTESIAN_POINT ( 'NONE',  ( -7.130211940009568927, -7.605417807865418212, 6.857782953271941950E-17 ) ) ;
#11843=CARTESIAN_POINT ( 'NONE',  ( -12.04643853703213807, -0.2059847383341459892, 10.00000000000000000 ) ) ;
#11847=CARTESIAN_POINT ( 'NONE',  ( -8.409270314015810044, 2.833341551407462244, 3.747395293195558847E-16 ) ) ;
#11861=CARTESIAN_POINT ( 'NONE',  ( 0.6279411196271849072, -4.781877258324066737, 6.857782953271941950E-17 ) ) ;
#11868=CARTESIAN_POINT ( 'NONE',  ( -0.9167995209625440234, 5.268308710424125074, 10.00000000000000000 ) ) ;
#11874=CARTESIAN_POINT ( 'NONE',  ( 5.027256439335601179, -9.798587832406491671, 10.00000000000000000 ) ) ;
#11882=CARTESIAN_POINT ( 'NONE',  ( 3.571029491936644540, 3.388293644658557646, 3.747395293195558847E-16 ) ) ;
#11891=CARTESIAN_POINT ( 'NONE',  ( -5.542557460684662374, -4.854674288180239827, 10.00000000000000000 ) ) ;
#11893=CARTESIAN_POINT ( 'NONE',  ( -5.125696908148159814, -9.212757455309411370, 6.857782953271941950E-17 ) ) ;
#11901=CARTESIAN_POINT ( 'NONE',  ( 7.019749797092301513, 12.16723183298456057, 10.00000000000000000 ) ) ;
#11906=CARTESIAN_POINT ( 'NONE',  ( -7.370305768634978882, 4.727533884956530486, 3.747395293195558847E-16 ) ) ;
#11919=CARTESIAN_POINT ( 'NONE',  ( 4.346347989803176937, 4.041826679702269942, 6.857782953271941950E-17 ) ) ;
#11928=CARTESIAN_POINT ( 'NONE',  ( -0.1881845630465191765, -6.755137126427050553, 10.00000000000000000 ) ) ;
#11934=CARTESIAN_POINT ( 'NONE',  ( -6.825012239887744414, 1.243808647927287403, 10.00000000000000000 ) ) ;
#11943=CARTESIAN_POINT ( 'NONE',  ( 0.5697670706242773386, -3.781298318517893442, 3.747395293195558847E-16 ) ) ;
#11952=CARTESIAN_POINT ( 'NONE',  ( -0.2556890074706221205, -7.756263830888991961, 6.857782953271941950E-17 ) ) ;
#11962=CARTESIAN_POINT ( 'NONE',  ( 10.44364468045616157, 9.157203537818526584, 10.00000000000000000 ) ) ;
#11967=CARTESIAN_POINT ( 'NONE',  ( 7.261170810407326037, -1.543028577657243439, 3.747395293195558847E-16 ) ) ;
#11984=CARTESIAN_POINT ( 'NONE',  ( 5.531377455021717182, -0.3672033614207537711, 6.857782953271941950E-17 ) ) ;
#11994=CARTESIAN_POINT ( 'NONE',  ( -5.359287035704432434, 6.724520318541068242, 10.00000000000000000 ) ) ;
#12002=CARTESIAN_POINT ( 'NONE',  ( -15.18624859168667562, -5.715447929355453205, 6.857782953271941950E-17 ) ) ;
#12009=CARTESIAN_POINT ( 'NONE',  ( 6.723006375386860967, 3.907299473125124489, 3.747395293195558847E-16 ) ) ;
#12012=EDGE_CURVE ( 'NONE', #3450, #4165, #161, .T. ) ;
#12017=CARTESIAN_POINT ( 'NONE',  ( 6.242895496888662521, -5.302832405932363713, 6.857782953271941950E-17 ) ) ;
#12023=CARTESIAN_POINT ( 'NONE',  ( -4.622662292628551661, -8.344572748942844953, 10.00000000000000000 ) ) ;
#12027=CARTESIAN_POINT ( 'NONE',  ( 0.6578947103914138950, -9.792230064638470566, 3.747395293195558847E-16 ) ) ;
#12028=CARTESIAN_POINT ( 'NONE',  ( 1.631735293711819246, 4.895207720155139164, 3.747395293195558847E-16 ) ) ;
#12042=CARTESIAN_POINT ( 'NONE',  ( 15.00667705184753764, -6.512453894250635145, 3.747395293195558847E-16 ) ) ;
#12043=CARTESIAN_POINT ( 'NONE',  ( 7.449730884303669143, -3.679036338562942543, 6.857782953271941950E-17 ) ) ;
#12052=CARTESIAN_POINT ( 'NONE',  ( 5.211919109253434712, 5.981019939437272726, 10.00000000000000000 ) ) ;
#12058=CARTESIAN_POINT ( 'NONE',  ( 14.52660474336492236, -9.366294961249355566, 6.857782953271941950E-17 ) ) ;
#12065=CARTESIAN_POINT ( 'NONE',  ( -5.704017324792769905, 1.489539271746818772, 3.747395293195558847E-16 ) ) ;
#12073=CARTESIAN_POINT ( 'NONE',  ( -3.764233030011069125, -6.516208816467297105, 6.857782953271941950E-17 ) ) ;
#12082=CARTESIAN_POINT ( 'NONE',  ( 8.800885721068839374, 6.316044917328129671, 10.00000000000000000 ) ) ;
#12086=CARTESIAN_POINT ( 'NONE',  ( -4.622662292628548997, -8.344572748942098883, 3.747395293195558847E-16 ) ) ;
#12099=CARTESIAN_POINT ( 'NONE',  ( 12.88139461472923841, -9.891864711284155121, 3.747395293195558847E-16 ) ) ;
#12100=CARTESIAN_POINT ( 'NONE',  ( -2.570438583093345386, 5.934334910739564428, 6.857782953271941950E-17 ) ) ;
#12107=ORIENTED_EDGE ( 'NONE', *, *, #5237, .F. ) ;
#12111=CARTESIAN_POINT ( 'NONE',  ( 4.516389116325776776, 1.247036727255508737, 10.00000000000000000 ) ) ;
ENDSEC;
END-ISO-10303-21;
